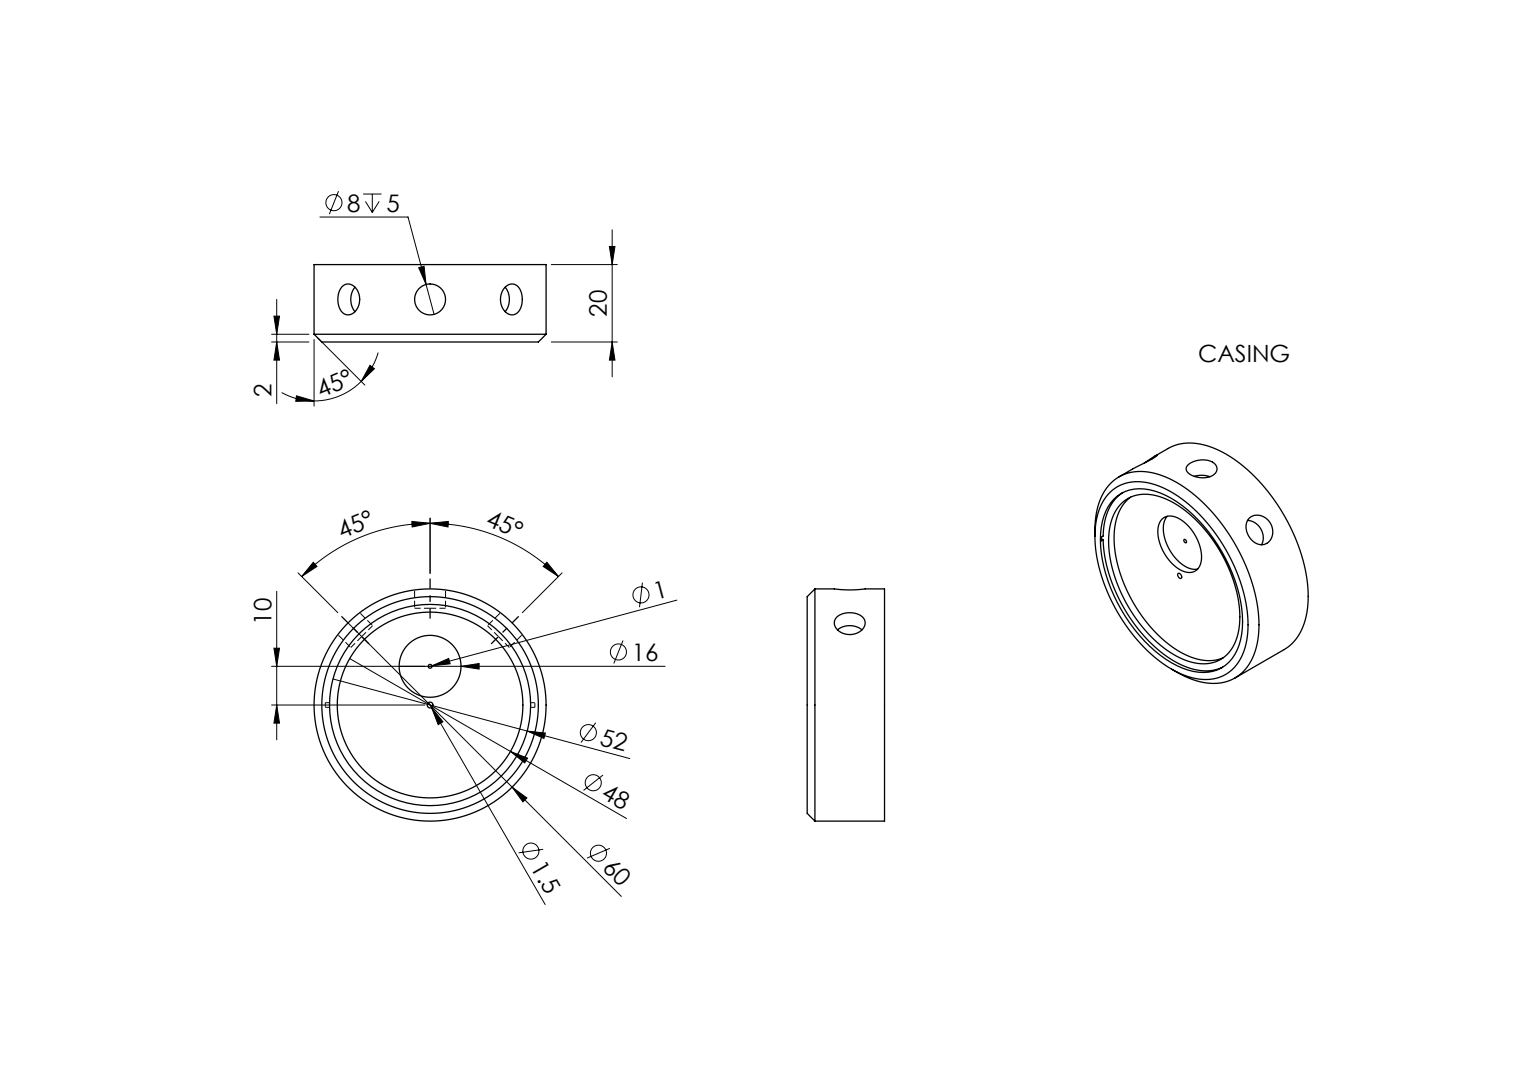
ISO-10303-21;
HEADER;
FILE_DESCRIPTION (('STEP AP214'),
    '1' );
FILE_NAME ('casing.step',
    '2026-10-26T11:20:31',
    ( '' ),
    ( '' ),
    'SwSTEP 2.0',
    'SolidWorks 2026',
    '' );
FILE_SCHEMA (( 'AUTOMOTIVE_DESIGN' ));
ENDSEC;

DATA;
#4=DIRECTION ( 'NONE',  ( 1.000000000000000000, 0.000000000000000000, 0.000000000000000000 ) ) ;
#15=CIRCLE ( 'NONE', #3506, 24.00000000000000355 ) ;
#17=CARTESIAN_POINT ( 'NONE',  ( 23.85222316637485562, 18.19536891688241198, 8.735393166554770161 ) ) ;
#23=EDGE_CURVE ( 'NONE', #3682, #3477, #99, .T. ) ;
#24=EDGE_CURVE ( 'NONE', #786, #1876, #1622, .T. ) ;
#31=CARTESIAN_POINT ( 'NONE',  ( -23.83674813237297130, 18.21571070649537916, 9.520895848189303123 ) ) ;
#33=CARTESIAN_POINT ( 'NONE',  ( -25.16843286583315376, -6.741346781237213648, 20.00001200000000168 ) ) ;
#38=CARTESIAN_POINT ( 'NONE',  ( 0.000000000000000000, 10.00000000000000000, 13.00000000000000178 ) ) ;
#40=CARTESIAN_POINT ( 'NONE',  ( 18.61772044889877264, 23.52449179749628883, 6.992605352578564748 ) ) ;
#41=CARTESIAN_POINT ( 'NONE',  ( -3.013274039476890653, 29.84885987243285399, 6.356496494711869616 ) ) ;
#43=MECHANICAL_DESIGN_GEOMETRIC_PRESENTATION_REPRESENTATION('',(#878),#2695);
#44=ORIENTED_EDGE ( 'NONE', *, *, #3267, .F. ) ;
#45=EDGE_CURVE ( 'NONE', #4134, #2111, #508, .T. ) ;
#57=LINE ( 'NONE', #2588, #2669 ) ;
#59=DIRECTION ( 'NONE',  ( 1.000000000000000000, 0.000000000000000000, 0.000000000000000000 ) ) ;
#64=CARTESIAN_POINT ( 'NONE',  ( 21.58020450303990145, 20.84134157445924274, 5.025533726064748130 ) ) ;
#69=ORIENTED_EDGE ( 'NONE', *, *, #4531, .T. ) ;
#72=AXIS2_PLACEMENT_3D ( 'NONE', #1710, #1001, #219 ) ;
#81=CARTESIAN_POINT ( 'NONE',  ( -18.19536891688249014, 23.85222316637480233, 9.264542937126581279 ) ) ;
#92=CARTESIAN_POINT ( 'NONE',  ( 23.23634976112698780, 18.97646788767667303, 6.355262957884884933 ) ) ;
#96=ORIENTED_EDGE ( 'NONE', *, *, #3914, .F. ) ;
#99=CIRCLE ( 'NONE', #4660, 24.00000000000000355 ) ;
#101=CYLINDRICAL_SURFACE ( 'NONE', #1304, 4.000000000000000000 ) ;
#105=EDGE_LOOP ( 'NONE', ( #1327, #855, #1076, #4619 ) ) ;
#107=CARTESIAN_POINT ( 'NONE',  ( -23.85222316637485207, 18.19536891688241553, 9.261144538644668245 ) ) ;
#108=CARTESIAN_POINT ( 'NONE',  ( 27.09999999999999787, -0.5999999999999998668, 19.59999999999999787 ) ) ;
#110=CARTESIAN_POINT ( 'NONE',  ( 27.09999999999999787, -0.5999999999999998668, 19.00000000000000000 ) ) ;
#111=CARTESIAN_POINT ( 'NONE',  ( 26.00000000000000355, 3.184081677783117796E-15, 19.59999999999999787 ) ) ;
#112=ADVANCED_FACE ( 'NONE', ( #3592 ), #4601, .T. ) ;
#115=CYLINDRICAL_SURFACE ( 'NONE', #1174, 24.00000000000000355 ) ;
#117=ORIENTED_EDGE ( 'NONE', *, *, #24, .F. ) ;
#122=AXIS2_PLACEMENT_3D ( 'NONE', #3838, #2369, #3476 ) ;
#125=ORIENTED_EDGE ( 'NONE', *, *, #1308, .T. ) ;
#126=EDGE_LOOP ( 'NONE', ( #4196, #3326, #979, #96 ) ) ;
#127=VERTEX_POINT ( 'NONE', #2121 ) ;
#131=VECTOR ( 'NONE', #4325, 1000.000000000000000 ) ;
#138=DIRECTION ( 'NONE',  ( 0.000000000000000000, -0.000000000000000000, -1.000000000000000000 ) ) ;
#143=DIRECTION ( 'NONE',  ( 1.000000000000000000, 0.000000000000000000, 0.000000000000000000 ) ) ;
#151=ORIENTED_EDGE ( 'NONE', *, *, #3914, .T. ) ;
#152=CARTESIAN_POINT ( 'NONE',  ( -25.99307600111999150, -0.5999999999999996447, 19.00000000000000000 ) ) ;
#157=CARTESIAN_POINT ( 'NONE',  ( -27.10000000000000497, -0.5999999999999998668, 19.00000000000000000 ) ) ;
#161=VECTOR ( 'NONE', #2341, 1000.000000000000000 ) ;
#162=CARTESIAN_POINT ( 'NONE',  ( -3.974466138550253103, 29.73560671006806899, 8.477544402765669673 ) ) ;
#164=PLANE ( 'NONE',  #630 ) ;
#169=EDGE_LOOP ( 'NONE', ( #4072, #812, #3404, #1028 ) ) ;
#171=EDGE_CURVE ( 'NONE', #2679, #1375, #2788, .T. ) ;
#174=PLANE ( 'NONE',  #3718 ) ;
#176=CIRCLE ( 'NONE', #3436, 4.000000000000000000 ) ;
#179=CARTESIAN_POINT ( 'NONE',  ( 0.000000000000000000, 10.00000000000000000, 15.00000000000000178 ) ) ;
#180=CARTESIAN_POINT ( 'NONE',  ( 8.000000000000000000, 10.00000000000000000, 15.00000000000000178 ) ) ;
#181=VERTEX_POINT ( 'NONE', #3190 ) ;
#185=CARTESIAN_POINT ( 'NONE',  ( -18.51903806033412891, 23.60202272616344743, 7.225073904196622543 ) ) ;
#187=CARTESIAN_POINT ( 'NONE',  ( -24.67207871933484498, 8.377607117416790317, 20.00001200000000523 ) ) ;
#189=EDGE_CURVE ( 'NONE', #2680, #3477, #311, .T. ) ;
#193=ADVANCED_FACE ( 'NONE', ( #334 ), #4702, .T. ) ;
#194=ORIENTED_EDGE ( 'NONE', *, *, #171, .F. ) ;
#195=CARTESIAN_POINT ( 'NONE',  ( 0.000000000000000000, 0.000000000000000000, 17.00000000000000000 ) ) ;
#204=EDGE_LOOP ( 'NONE', ( #2319, #1799, #3397, #669 ) ) ;
#208=CARTESIAN_POINT ( 'NONE',  ( 19.74742367678139132, 22.58509718322848769, 12.47015313278852844 ) ) ;
#212=CARTESIAN_POINT ( 'NONE',  ( -13.02991752792604707, 22.56362157461192908, 20.00001199999999812 ) ) ;
#217=ORIENTED_EDGE ( 'NONE', *, *, #23, .F. ) ;
#219=DIRECTION ( 'NONE',  ( 1.000000000000000000, 0.000000000000000000, 0.000000000000000000 ) ) ;
#220=DIRECTION ( 'NONE',  ( 0.000000000000000000, 0.000000000000000000, -1.000000000000000000 ) ) ;
#221=DIRECTION ( 'NONE',  ( 0.000000000000000000, 0.000000000000000000, 1.000000000000000000 ) ) ;
#224=CARTESIAN_POINT ( 'NONE',  ( 0.000000000000000000, 10.00000000000000000, 13.00000000000000178 ) ) ;
#226=FACE_OUTER_BOUND ( 'NONE', #2584, .T. ) ;
#227=EDGE_CURVE ( 'NONE', #883, #4468, #2767, .T. ) ;
#230=EDGE_CURVE ( 'NONE', #2552, #3925, #639, .T. ) ;
#236=DIRECTION ( 'NONE',  ( 0.000000000000000000, 0.000000000000000000, 1.000000000000000000 ) ) ;
#238=ORIENTED_EDGE ( 'NONE', *, *, #407, .F. ) ;
#239=EDGE_LOOP ( 'NONE', ( #2558, #2162, #259, #4443, #4049, #3898, #2909, #3068 ) ) ;
#240=FACE_OUTER_BOUND ( 'NONE', #4032, .T. ) ;
#241=DIRECTION ( 'NONE',  ( 0.000000000000000000, 0.000000000000000000, 1.000000000000000000 ) ) ;
#242=CARTESIAN_POINT ( 'NONE',  ( -3.403349963601461248, 25.83240171513484285, 20.00001200000000168 ) ) ;
#245=LINE ( 'NONE', #1716, #3549 ) ;
#247=VECTOR ( 'NONE', #3763, 1000.000000000000000 ) ;
#251=CARTESIAN_POINT ( 'NONE',  ( 18.51766120599535981, 23.60309964903844104, 10.77116693461329078 ) ) ;
#254=ADVANCED_FACE ( 'NONE', ( #2730 ), #1312, .F. ) ;
#259=ORIENTED_EDGE ( 'NONE', *, *, #1804, .T. ) ;
#262=FACE_OUTER_BOUND ( 'NONE', #1955, .T. ) ;
#265=SURFACE_SIDE_STYLE ('',( #3589 ) ) ;
#266=CARTESIAN_POINT ( 'NONE',  ( 27.09999999999999787, -0.5999999999999998668, 19.59999999999999787 ) ) ;
#268=AXIS2_PLACEMENT_3D ( 'NONE', #458, #2589, #3308 ) ;
#271=CARTESIAN_POINT ( 'NONE',  ( 0.2611446086310952874, 29.99999999999999645, 12.99999999999999112 ) ) ;
#272=ORIENTED_EDGE ( 'NONE', *, *, #761, .F. ) ;
#275=DIRECTION ( 'NONE',  ( 0.000000000000000000, 0.000000000000000000, 1.000000000000000000 ) ) ;
#276=CARTESIAN_POINT ( 'NONE',  ( 0.7500000000000001110, 0.000000000000000000, 17.00000000000000000 ) ) ;
#278=CARTESIAN_POINT ( 'NONE',  ( 17.67766952966372429, 17.67766952966365679, 8.999999999999992895 ) ) ;
#280=FACE_OUTER_BOUND ( 'NONE', #719, .T. ) ;
#283=EDGE_CURVE ( 'NONE', #741, #1146, #1292, .T. ) ;
#284=ORIENTED_EDGE ( 'NONE', *, *, #1600, .T. ) ;
#287=SHAPE_REPRESENTATION_RELATIONSHIP ( 'NONE' , 'NONE' ,  #1408, #2500 ) ;
#289=VERTEX_POINT ( 'NONE', #3854 ) ;
#290=DIRECTION ( 'NONE',  ( -1.000000000000000000, 0.000000000000000000, 0.000000000000000000 ) ) ;
#295=CARTESIAN_POINT ( 'NONE',  ( 1.289767132401806071, 29.97323123820465440, 12.79530979536915858 ) ) ;
#299=CARTESIAN_POINT ( 'NONE',  ( 25.99307600111999150, -0.5999999999999996447, 19.00000000000000000 ) ) ;
#300=CARTESIAN_POINT ( 'NONE',  ( 25.83240171513484285, -3.403349963601437267, 20.00001200000000168 ) ) ;
#301=CARTESIAN_POINT ( 'NONE',  ( -22.58496929628987360, 19.74756467586668762, 5.529782636833617815 ) ) ;
#305=VERTEX_POINT ( 'NONE', #1266 ) ;
#309=EDGE_CURVE ( 'NONE', #2969, #127, #2118, .T. ) ;
#311=LINE ( 'NONE', #4676, #943 ) ;
#315=CARTESIAN_POINT ( 'NONE',  ( 1.037548646792561202, 29.98316644498967776, 12.87206112426449955 ) ) ;
#318=AXIS2_PLACEMENT_3D ( 'NONE', #3626, #2522, #799 ) ;
#321=CARTESIAN_POINT ( 'NONE',  ( -26.00000000000000355, -1.592040838891558504E-15, 20.00000599999999906 ) ) ;
#332=ADVANCED_FACE ( 'NONE', ( #1356 ), #2431, .F. ) ;
#334=FACE_OUTER_BOUND ( 'NONE', #3811, .T. ) ;
#336=DIRECTION ( 'NONE',  ( 0.7071067811865487940, -0.7071067811865463515, 0.000000000000000000 ) ) ;
#338=CARTESIAN_POINT ( 'NONE',  ( 0.000000000000000000, 0.000000000000000000, 17.00000000000000000 ) ) ;
#339=CARTESIAN_POINT ( 'NONE',  ( 2.445228802079471908, 29.90098466201939331, 5.823513562339502236 ) ) ;
#340=AXIS2_PLACEMENT_3D ( 'NONE', #4186, #2765, #968 ) ;
#343=CARTESIAN_POINT ( 'NONE',  ( 22.99946665860936079, 19.26288713789788076, 12.01444203287436174 ) ) ;
#350=ORIENTED_EDGE ( 'NONE', *, *, #987, .F. ) ;
#351=EDGE_LOOP ( 'NONE', ( #3080, #1048, #1376, #4284 ) ) ;
#353=DIRECTION ( 'NONE',  ( 0.000000000000000000, 0.000000000000000000, 1.000000000000000000 ) ) ;
#354=ORIENTED_EDGE ( 'NONE', *, *, #189, .T. ) ;
#360=VECTOR ( 'NONE', #3662, 1000.000000000000000 ) ;
#363=EDGE_CURVE ( 'NONE', #3116, #786, #4257, .T. ) ;
#365=CIRCLE ( 'NONE', #72, 0.5000000000000001110 ) ;
#368=AXIS2_PLACEMENT_3D ( 'NONE', #485, #3386, #138 ) ;
#373=DIRECTION ( 'NONE',  ( 0.000000000000000000, 0.000000000000000000, 1.000000000000000000 ) ) ;
#383=EDGE_LOOP ( 'NONE', ( #2433, #2317, #125, #4259 ) ) ;
#388=CARTESIAN_POINT ( 'NONE',  ( 23.60202272616350783, 18.51903806033405075, 7.225073904196623431 ) ) ;
#390=EDGE_CURVE ( 'NONE', #3925, #1876, #667, .T. ) ;
#392=ADVANCED_FACE ( 'NONE', ( #280 ), #3556, .F. ) ;
#394=ORIENTED_EDGE ( 'NONE', *, *, #1600, .F. ) ;
#401=ORIENTED_EDGE ( 'NONE', *, *, #3956, .F. ) ;
#405=FACE_OUTER_BOUND ( 'NONE', #3345, .T. ) ;
#406=DIRECTION ( 'NONE',  ( -0.000000000000000000, -0.000000000000000000, 1.000000000000000000 ) ) ;
#407=EDGE_CURVE ( 'NONE', #4099, #956, #3629, .T. ) ;
#409=AXIS2_PLACEMENT_3D ( 'NONE', #952, #3826, #4194 ) ;
#414=CARTESIAN_POINT ( 'NONE',  ( 22.43029000766442493, 19.92335677698576291, 5.404794703904384434 ) ) ;
#417=EDGE_LOOP ( 'NONE', ( #3095, #2362, #3318, #3383, #3652 ) ) ;
#421=AXIS2_PLACEMENT_3D ( 'NONE', #2479, #3250, #1065 ) ;
#431=CARTESIAN_POINT ( 'NONE',  ( -23.77376218378628181, 18.29783893517727478, 10.03754308049874311 ) ) ;
#433=CARTESIAN_POINT ( 'NONE',  ( 26.00000000000000355, 1.592040838891558898E-15, 20.00000599999999906 ) ) ;
#436=CYLINDRICAL_SURFACE ( 'NONE', #571, 3.999999999999998224 ) ;
#452=ORIENTED_EDGE ( 'NONE', *, *, #2236, .F. ) ;
#458=CARTESIAN_POINT ( 'NONE',  ( 0.000000000000000000, 10.00000000000000000, 15.00000000000000178 ) ) ;
#462=CARTESIAN_POINT ( 'NONE',  ( -27.10000000000000497, -0.5999999999999998668, 19.59999999999999787 ) ) ;
#465=CARTESIAN_POINT ( 'NONE',  ( 0.000000000000000000, 0.000000000000000000, 17.99999999999998579 ) ) ;
#470=CARTESIAN_POINT ( 'NONE',  ( -17.67766952966371719, 17.67766952966366389, 8.999999999999992895 ) ) ;
#471=CARTESIAN_POINT ( 'NONE',  ( -27.10000000000000497, -0.5999999999999998668, 19.00000000000000000 ) ) ;
#476=ORIENTED_EDGE ( 'NONE', *, *, #1700, .F. ) ;
#480=CARTESIAN_POINT ( 'NONE',  ( -18.61790092284054410, 23.52435923723752609, 11.00811882721853152 ) ) ;
#485=CARTESIAN_POINT ( 'NONE',  ( -27.10000000000000497, 0.6000000000000000888, 19.59999999999999787 ) ) ;
#490=CARTESIAN_POINT ( 'NONE',  ( -1.774938052278379752, 29.94842879300231075, 5.405792698933810314 ) ) ;
#500=ORIENTED_EDGE ( 'NONE', *, *, #1073, .F. ) ;
#501=ORIENTED_EDGE ( 'NONE', *, *, #866, .F. ) ;
#506=CARTESIAN_POINT ( 'NONE',  ( 0.000000000000000000, 0.000000000000000000, 17.00000000000000000 ) ) ;
#508=LINE ( 'NONE', #3408, #1317 ) ;
#513=ORIENTED_EDGE ( 'NONE', *, *, #1744, .T. ) ;
#519=CARTESIAN_POINT ( 'NONE',  ( -18.29773070266338664, 23.77384460521234288, 7.963596978677149885 ) ) ;
#533=ORIENTED_EDGE ( 'NONE', *, *, #4639, .F. ) ;
#534=DIRECTION ( 'NONE',  ( 0.000000000000000000, 1.000000000000000000, 0.000000000000000000 ) ) ;
#535=PLANE ( 'NONE',  #4253 ) ;
#536=FACE_BOUND ( 'NONE', #2532, .T. ) ;
#537=ORIENTED_EDGE ( 'NONE', *, *, #1804, .F. ) ;
#539=VECTOR ( 'NONE', #2025, 1000.000000000000000 ) ;
#540=CARTESIAN_POINT ( 'NONE',  ( 18.19536891688249369, 23.85222316637479523, 8.999999999999992895 ) ) ;
#547=DIRECTION ( 'NONE',  ( 1.000000000000000000, 0.000000000000000000, 0.000000000000000000 ) ) ;
#549=EDGE_LOOP ( 'NONE', ( #476, #1269 ) ) ;
#550=ORIENTED_EDGE ( 'NONE', *, *, #3857, .F. ) ;
#561=ORIENTED_EDGE ( 'NONE', *, *, #1435, .T. ) ;
#567=CARTESIAN_POINT ( 'NONE',  ( -18.61638332444503519, 23.52555220673917447, 6.995423750305947763 ) ) ;
#569=CARTESIAN_POINT ( 'NONE',  ( -26.00000000000000355, -1.592040838891558504E-15, 20.00000599999999906 ) ) ;
#571=AXIS2_PLACEMENT_3D ( 'NONE', #3387, #3314, #1154 ) ;
#585=DIRECTION ( 'NONE',  ( 0.000000000000000000, 0.000000000000000000, 1.000000000000000000 ) ) ;
#586=CARTESIAN_POINT ( 'NONE',  ( 3.469446951953614189E-15, 30.00000000000000355, 8.999999999999992895 ) ) ;
#591=CARTESIAN_POINT ( 'NONE',  ( -14.84924240491753089, 20.50609665440985552, 8.999999999999992895 ) ) ;
#593=CARTESIAN_POINT ( 'NONE',  ( 19.25985638980603554, 23.00200370561274354, 12.01100206247544300 ) ) ;
#594=DIRECTION ( 'NONE',  ( -1.000000000000000000, -0.000000000000000000, -0.000000000000000000 ) ) ;
#595=CARTESIAN_POINT ( 'NONE',  ( -21.58204166899923138, 20.83941891177991224, 5.025993266704736229 ) ) ;
#602=CARTESIAN_POINT ( 'NONE',  ( -27.10000000000000497, 0.6000000000000000888, 19.59999999999999787 ) ) ;
#606=STYLED_ITEM('',(#4736),#2883);
#611=EDGE_CURVE ( 'NONE', #4468, #4460, #1182, .T. ) ;
#616=CARTESIAN_POINT ( 'NONE',  ( -2.007411586324088226, 29.93355017142139118, 12.46960170373642640 ) ) ;
#618=CARTESIAN_POINT ( 'NONE',  ( -23.85222316637485562, 18.19536891688241198, 8.999999999999992895 ) ) ;
#623=ORIENTED_EDGE ( 'NONE', *, *, #3700, .F. ) ;
#624=ADVANCED_FACE ( 'NONE', ( #2648 ), #2287, .T. ) ;
#629=CARTESIAN_POINT ( 'NONE',  ( 8.377607117416813409, 24.67207871933482366, 20.00001200000000523 ) ) ;
#630=AXIS2_PLACEMENT_3D ( 'NONE', #850, #2727, #2290 ) ;
#634=CARTESIAN_POINT ( 'NONE',  ( 3.796098697355190676, 29.75902942016942987, 7.712254142552557923 ) ) ;
#639=CIRCLE ( 'NONE', #3339, 26.00000000000000355 ) ;
#640=DIRECTION ( 'NONE',  ( 0.000000000000000000, 0.000000000000000000, -1.000000000000000000 ) ) ;
#644=DIRECTION ( 'NONE',  ( 1.000000000000000000, 0.000000000000000000, 0.000000000000000000 ) ) ;
#647=CIRCLE ( 'NONE', #3292, 26.00000000000000355 ) ;
#648=CARTESIAN_POINT ( 'NONE',  ( 27.09999999999999787, 0.6000000000000000888, 19.59999999999999787 ) ) ;
#649=DIRECTION ( 'NONE',  ( 0.000000000000000000, 0.000000000000000000, -1.000000000000000000 ) ) ;
#650=CIRCLE ( 'NONE', #4445, 26.00000000000000355 ) ;
#651=( LENGTH_UNIT ( ) NAMED_UNIT ( * ) SI_UNIT ( .MILLI., .METRE. ) );
#656=( GEOMETRIC_REPRESENTATION_CONTEXT ( 3 ) GLOBAL_UNCERTAINTY_ASSIGNED_CONTEXT ( ( #1169 ) ) GLOBAL_UNIT_ASSIGNED_CONTEXT ( ( #3518, #1074, #4331 ) ) REPRESENTATION_CONTEXT ( 'NONE', 'WORKASPACE' ) );
#657=( NAMED_UNIT ( * ) SI_UNIT ( $, .STERADIAN. ) SOLID_ANGLE_UNIT ( ) );
#665=CARTESIAN_POINT ( 'NONE',  ( -23.52449179749635277, 18.61772044889870159, 6.992605352578565636 ) ) ;
#667=LINE ( 'NONE', #1046, #131 ) ;
#669=ORIENTED_EDGE ( 'NONE', *, *, #1744, .F. ) ;
#674=CARTESIAN_POINT ( 'NONE',  ( 24.00000000000000355, 0.000000000000000000, 17.00000000000000000 ) ) ;
#679=DIRECTION ( 'NONE',  ( 1.000000000000000000, 0.000000000000000000, 0.000000000000000000 ) ) ;
#681=CYLINDRICAL_SURFACE ( 'NONE', #1102, 0.7500000000000001110 ) ;
#694=ORIENTED_EDGE ( 'NONE', *, *, #4339, .F. ) ;
#698=VECTOR ( 'NONE', #1121, 1000.000000000000000 ) ;
#703=LINE ( 'NONE', #1079, #900 ) ;
#704=CARTESIAN_POINT ( 'NONE',  ( 3.872997316437435167, 29.74899170013632954, 7.966596725458382267 ) ) ;
#705=CIRCLE ( 'NONE', #1311, 0.7500000000000001110 ) ;
#707=VECTOR ( 'NONE', #1175, 1000.000000000000000 ) ;
#708=B_SPLINE_CURVE_WITH_KNOTS ( 'NONE', 3,
 ( #3293, #846, #2286, #1159, #3745, #490, #823, #2264, #4490, #41, #2216, #1864, #3670, #1604, #4165, #162, #3129, #3463, #2745, #2796, #4252, #2351, #4610, #898, #2425, #2037, #3823, #616, #2328, #1989, #993, #948, #2770, #3438 ),
 .UNSPECIFIED., .F., .F.,
 ( 4, 2, 2, 2, 2, 2, 2, 2, 2, 2, 2, 2, 2, 2, 2, 2, 4 ),
 ( 0.000000000000000000, 0.0007824850735655043557, 0.001564970147131008711, 0.002347455220696513176, 0.003129940294262017423, 0.003912425367827521670, 0.004694910441393026351, 0.005477395514958530165, 0.006259880588524034846, 0.007042365662089539527, 0.007824850735655043341, 0.008607335809220547154, 0.009389820882786052703, 0.01017230595635155652, 0.01095479102991706033, 0.01173727610348256588, 0.01251976117704806969 ),
 .UNSPECIFIED. ) ;
#712=CARTESIAN_POINT ( 'NONE',  ( -27.10000000000000497, -0.5999999999999998668, 19.00000000000000000 ) ) ;
#719=EDGE_LOOP ( 'NONE', ( #3325, #1461, #3259, #694 ) ) ;
#721=CARTESIAN_POINT ( 'NONE',  ( 3.403349963601422168, 25.83240171513484285, 20.00001200000000523 ) ) ;
#722=EDGE_CURVE ( 'NONE', #4523, #3514, #2026, .T. ) ;
#724=EDGE_CURVE ( 'NONE', #2854, #2731, #4586, .T. ) ;
#729=AXIS2_PLACEMENT_3D ( 'NONE', #506, #221, #3815 ) ;
#730=DIRECTION ( 'NONE',  ( 1.000000000000000000, 0.000000000000000000, -0.000000000000000000 ) ) ;
#731=CIRCLE ( 'NONE', #3389, 8.000000000000000000 ) ;
#732=CYLINDRICAL_SURFACE ( 'NONE', #3891, 0.7500000000000001110 ) ;
#735=VECTOR ( 'NONE', #2831, 1000.000000000000000 ) ;
#740=DIRECTION ( 'NONE',  ( 1.000000000000000000, 0.000000000000000000, 0.000000000000000000 ) ) ;
#741=VERTEX_POINT ( 'NONE', #2403 ) ;
#747=EDGE_LOOP ( 'NONE', ( #2220, #2706, #1118, #1381 ) ) ;
#749=EDGE_CURVE ( 'NONE', #1146, #1098, #2012, .T. ) ;
#750=VECTOR ( 'NONE', #3405, 1000.000000000000000 ) ;
#761=EDGE_CURVE ( 'NONE', #4484, #1375, #3922, .T. ) ;
#769=CARTESIAN_POINT ( 'NONE',  ( -18.84808613845423508, 23.34033764136069422, 11.44520879210846687 ) ) ;
#770=DIRECTION ( 'NONE',  ( -0.000000000000000000, -0.000000000000000000, -1.000000000000000000 ) ) ;
#771=CARTESIAN_POINT ( 'NONE',  ( 15.85973458909327505, -20.67279826512041296, 20.00001199999999457 ) ) ;
#772=ORIENTED_EDGE ( 'NONE', *, *, #1404, .T. ) ;
#775=CARTESIAN_POINT ( 'NONE',  ( -8.000000000000000000, 10.00000000000000178, 15.00000000000000178 ) ) ;
#778=EDGE_CURVE ( 'NONE', #956, #1513, #731, .T. ) ;
#779=DIRECTION ( 'NONE',  ( -0.000000000000000000, -0.000000000000000000, 1.000000000000000000 ) ) ;
#786=VERTEX_POINT ( 'NONE', #4232 ) ;
#789=DIRECTION ( 'NONE',  ( -0.000000000000000000, -0.000000000000000000, 1.000000000000000000 ) ) ;
#793=EDGE_LOOP ( 'NONE', ( #1095, #3584 ) ) ;
#794=AXIS2_PLACEMENT_3D ( 'NONE', #465, #2986, #2671 ) ;
#796=DIRECTION ( 'NONE',  ( 1.000000000000000000, 0.000000000000000000, 0.000000000000000000 ) ) ;
#797=AXIS2_PLACEMENT_3D ( 'NONE', #4318, #1787, #3597 ) ;
#799=DIRECTION ( 'NONE',  ( 1.000000000000000000, 0.000000000000000000, 0.000000000000000000 ) ) ;
#802=ORIENTED_EDGE ( 'NONE', *, *, #1661, .F. ) ;
#811=ORIENTED_EDGE ( 'NONE', *, *, #4287, .T. ) ;
#812=ORIENTED_EDGE ( 'NONE', *, *, #1517, .F. ) ;
#814=CARTESIAN_POINT ( 'NONE',  ( -21.40213195504977861, 21.02424009228906243, 12.99981531858142425 ) ) ;
#817=CARTESIAN_POINT ( 'NONE',  ( -25.99307600111999150, 0.5999999999999998668, 19.59999999999999787 ) ) ;
#822=CARTESIAN_POINT ( 'NONE',  ( 18.19536891688249369, 23.85222316637479523, 8.999999999999992895 ) ) ;
#823=CARTESIAN_POINT ( 'NONE',  ( -2.004590926901224535, 29.93374515888019971, 5.528701699505815803 ) ) ;
#830=DIRECTION ( 'NONE',  ( 1.000000000000000000, 0.000000000000000000, 0.000000000000000000 ) ) ;
#840=CARTESIAN_POINT ( 'NONE',  ( -23.00200370561280749, 19.25985638980596093, 12.01100206247544300 ) ) ;
#843=AXIS2_PLACEMENT_3D ( 'NONE', #2460, #2508, #3928 ) ;
#846=CARTESIAN_POINT ( 'NONE',  ( -0.2646063747045178660, 30.00000000000000000, 4.999999999999992895 ) ) ;
#850=CARTESIAN_POINT ( 'NONE',  ( -27.10000000000000497, -0.5999999999999998668, 19.59999999999999787 ) ) ;
#855=ORIENTED_EDGE ( 'NONE', *, *, #2538, .T. ) ;
#866=EDGE_CURVE ( 'NONE', #4468, #883, #1530, .T. ) ;
#867=DIRECTION ( 'NONE',  ( 0.000000000000000000, 0.000000000000000000, 1.000000000000000000 ) ) ;
#869=ORIENTED_EDGE ( 'NONE', *, *, #722, .T. ) ;
#871=B_SPLINE_CURVE_WITH_KNOTS ( 'NONE', 3,
 ( #540, #1305, #4536, #1281, #4211, #251, #1652, #1969, #1353, #593, #3416, #208, #2011, #2724, #3109, #2376, #3847, #1330, #4231, #3870, #1698, #1085, #4341, #3986, #343, #1745, #2911, #4635, #2104, #2520, #1722, #3624, #2497, #3529 ),
 .UNSPECIFIED., .F., .F.,
 ( 4, 2, 2, 2, 2, 2, 2, 2, 2, 2, 2, 2, 2, 2, 2, 2, 4 ),
 ( 0.01251975318912558477, 0.01330204881184919585, 0.01408434443457280694, 0.01486664005729641802, 0.01564893568002002910, 0.01643123130274364019, 0.01721352692546725127, 0.01799582254819086236, 0.01877811817091447344, 0.01956041379363808452, 0.02034270941636169561, 0.02112500503908530669, 0.02190730066180891430, 0.02268959628453252539, 0.02347189190725613647, 0.02425418752997974756, 0.02503648315270335864 ),
 .UNSPECIFIED. ) ;
#875=CARTESIAN_POINT ( 'NONE',  ( -20.46659425767094120, 21.93593546006592732, 5.128325996195414405 ) ) ;
#878=STYLED_ITEM ( 'NONE', ( #1424 ), #2500 ) ;
#879=DIRECTION ( 'NONE',  ( 0.000000000000000000, -1.000000000000000000, 0.000000000000000000 ) ) ;
#882=ORIENTED_EDGE ( 'NONE', *, *, #3578, .T. ) ;
#883=VERTEX_POINT ( 'NONE', #433 ) ;
#884=CARTESIAN_POINT ( 'NONE',  ( 0.000000000000000000, 0.000000000000000000, 20.00000000000000000 ) ) ;
#891=ADVANCED_FACE ( 'NONE', ( #1883 ), #3893, .F. ) ;
#893=FACE_BOUND ( 'NONE', #793, .T. ) ;
#897=EDGE_CURVE ( 'NONE', #1997, #4134, #2797, .T. ) ;
#898=CARTESIAN_POINT ( 'NONE',  ( -3.180741987853693331, 29.83126030492351788, 11.43940974718624837 ) ) ;
#900=VECTOR ( 'NONE', #4268, 1000.000000000000000 ) ;
#902=AXIS2_PLACEMENT_3D ( 'NONE', #2490, #3214, #3962 ) ;
#903=DIRECTION ( 'NONE',  ( -0.7071067811865487940, -0.7071067811865463515, 0.000000000000000000 ) ) ;
#906=VERTEX_POINT ( 'NONE', #3530 ) ;
#907=VERTEX_POINT ( 'NONE', #276 ) ;
#910=CARTESIAN_POINT ( 'NONE',  ( 3.959305739469038251E-15, 30.00000000000000355, 12.99999999999999289 ) ) ;
#913=DIRECTION ( 'NONE',  ( 0.000000000000000000, 0.000000000000000000, -1.000000000000000000 ) ) ;
#914=ADVANCED_FACE ( 'NONE', ( #4637 ), #2820, .F. ) ;
#930=CARTESIAN_POINT ( 'NONE',  ( -30.00000000000004974, 29.99999999999995737, 8.999999999999992895 ) ) ;
#943=VECTOR ( 'NONE', #1692, 1000.000000000000000 ) ;
#944=DIRECTION ( 'NONE',  ( 0.7071067811865487940, -0.7071067811865463515, 0.000000000000000000 ) ) ;
#948=CARTESIAN_POINT ( 'NONE',  ( -0.5265545572341292502, 29.99647701088549923, 12.97381592328244082 ) ) ;
#950=CIRCLE ( 'NONE', #3602, 8.000000000000000000 ) ;
#952=CARTESIAN_POINT ( 'NONE',  ( -17.67766952966371719, 17.67766952966366389, 8.999999999999992895 ) ) ;
#953=DIRECTION ( 'NONE',  ( 0.7071067811865462405, 0.7071067811865487940, 0.000000000000000000 ) ) ;
#956=VERTEX_POINT ( 'NONE', #1781 ) ;
#965=ORIENTED_EDGE ( 'NONE', *, *, #4384, .T. ) ;
#968=DIRECTION ( 'NONE',  ( 1.000000000000000000, 0.000000000000000000, -0.000000000000000000 ) ) ;
#974=EDGE_CURVE ( 'NONE', #127, #2969, #1720, .T. ) ;
#977=CARTESIAN_POINT ( 'NONE',  ( -27.99999999999999645, 0.000000000000000000, 20.00000000000000000 ) ) ;
#978=CARTESIAN_POINT ( 'NONE',  ( -26.00000000000000000, 1.701696020694461131, 20.00001199999999812 ) ) ;
#979=ORIENTED_EDGE ( 'NONE', *, *, #4589, .T. ) ;
#984=FILL_AREA_STYLE ('',( #1004 ) ) ;
#987=EDGE_CURVE ( 'NONE', #2090, #3682, #1802, .T. ) ;
#988=DIRECTION ( 'NONE',  ( 1.000000000000000000, 0.000000000000000000, 0.000000000000000000 ) ) ;
#991=CARTESIAN_POINT ( 'NONE',  ( 3.593167859435787204, 29.78421435497087444, 10.77704851721127177 ) ) ;
#993=CARTESIAN_POINT ( 'NONE',  ( -1.039771317798496408, 29.98307469845295969, 12.87134967428165666 ) ) ;
#994=CARTESIAN_POINT ( 'NONE',  ( -27.10000000000000497, -0.5999999999999998668, 19.59999999999999787 ) ) ;
#1001=DIRECTION ( 'NONE',  ( 0.000000000000000000, 0.000000000000000000, 1.000000000000000000 ) ) ;
#1004=FILL_AREA_STYLE_COLOUR ( '', #1477 ) ;
#1005=CARTESIAN_POINT ( 'NONE',  ( -6.741346781237239405, 25.16843286583313954, 20.00001200000000168 ) ) ;
#1009=CARTESIAN_POINT ( 'NONE',  ( 1.042990544031788813, 29.98297896446152322, 5.129385753419673399 ) ) ;
#1014=DIRECTION ( 'NONE',  ( -1.000000000000000000, 0.000000000000000000, 0.000000000000000000 ) ) ;
#1016=CARTESIAN_POINT ( 'NONE',  ( 13.02991752792604174, -22.56362157461193263, 20.00001200000000168 ) ) ;
#1017=CARTESIAN_POINT ( 'NONE',  ( -23.85222316637485562, 18.19536891688241909, 8.738792385868096702 ) ) ;
#1028=ORIENTED_EDGE ( 'NONE', *, *, #1435, .F. ) ;
#1031=CYLINDRICAL_SURFACE ( 'NONE', #3057, 0.5000000000000001110 ) ;
#1033=CARTESIAN_POINT ( 'NONE',  ( 3.472993751331377332, 29.79865100271689471, 6.998343904161816731 ) ) ;
#1034=EDGE_CURVE ( 'NONE', #181, #289, #4312, .T. ) ;
#1035=EDGE_CURVE ( 'NONE', #2995, #4460, #2546, .T. ) ;
#1042=CARTESIAN_POINT ( 'NONE',  ( 19.58805710660147170, -17.18149551509900519, 20.00001200000000523 ) ) ;
#1046=CARTESIAN_POINT ( 'NONE',  ( -27.10000000000000497, -0.5999999999999998668, 19.00000000000000000 ) ) ;
#1048=ORIENTED_EDGE ( 'NONE', *, *, #4587, .T. ) ;
#1049=CARTESIAN_POINT ( 'NONE',  ( -27.10000000000000497, 0.6000000000000000888, 19.59999999999999787 ) ) ;
#1052=ORIENTED_EDGE ( 'NONE', *, *, #749, .F. ) ;
#1055=FACE_OUTER_BOUND ( 'NONE', #1448, .T. ) ;
#1064=LINE ( 'NONE', #2194, #2300 ) ;
#1065=DIRECTION ( 'NONE',  ( 1.000000000000000000, 0.000000000000000000, 0.000000000000000000 ) ) ;
#1069=AXIS2_PLACEMENT_3D ( 'NONE', #4115, #2357, #1284 ) ;
#1073=EDGE_CURVE ( 'NONE', #3706, #3924, #2200, .T. ) ;
#1074=( NAMED_UNIT ( * ) PLANE_ANGLE_UNIT ( ) SI_UNIT ( $, .RADIAN. ) );
#1076=ORIENTED_EDGE ( 'NONE', *, *, #2773, .F. ) ;
#1077=CARTESIAN_POINT ( 'NONE',  ( 15.85973458909325728, 20.67279826512042362, 20.00001200000000168 ) ) ;
#1079=CARTESIAN_POINT ( 'NONE',  ( -27.10000000000000497, 0.6000000000000000888, 19.00000000000000000 ) ) ;
#1085=CARTESIAN_POINT ( 'NONE',  ( 22.42982507849026064, 19.92389804225921068, 12.59566700906149173 ) ) ;
#1088=DIRECTION ( 'NONE',  ( -0.000000000000000000, -0.000000000000000000, 1.000000000000000000 ) ) ;
#1093=PLANE ( 'NONE',  #3890 ) ;
#1095=ORIENTED_EDGE ( 'NONE', *, *, #3106, .F. ) ;
#1098=VERTEX_POINT ( 'NONE', #1901 ) ;
#1102=AXIS2_PLACEMENT_3D ( 'NONE', #3571, #2494, #4338 ) ;
#1104=DIRECTION ( 'NONE',  ( -0.000000000000000000, -0.000000000000000000, -1.000000000000000000 ) ) ;
#1107=AXIS2_PLACEMENT_3D ( 'NONE', #4548, #3049, #2713 ) ;
#1109=SHAPE_DEFINITION_REPRESENTATION ( #3051, #1408 ) ;
#1118=ORIENTED_EDGE ( 'NONE', *, *, #2395, .T. ) ;
#1121=DIRECTION ( 'NONE',  ( 0.7071067811865456854, 8.659560562354910671E-17, -0.7071067811865493491 ) ) ;
#1125=CARTESIAN_POINT ( 'NONE',  ( 25.99307600111999150, 0.6000000000000000888, 20.00001200000000168 ) ) ;
#1128=CARTESIAN_POINT ( 'NONE',  ( -22.56362157461193618, -13.02991752792603641, 20.00001200000000168 ) ) ;
#1135=AXIS2_PLACEMENT_3D ( 'NONE', #3491, #236, #3136 ) ;
#1137=CARTESIAN_POINT ( 'NONE',  ( 18.84534098761077914, 23.34254382248196791, 6.559627254860783019 ) ) ;
#1143=CARTESIAN_POINT ( 'NONE',  ( 0.000000000000000000, 0.000000000000000000, 17.00000000000000000 ) ) ;
#1146=VERTEX_POINT ( 'NONE', #3349 ) ;
#1147=ORIENTED_EDGE ( 'NONE', *, *, #45, .T. ) ;
#1149=LINE ( 'NONE', #1125, #4279 ) ;
#1151=CARTESIAN_POINT ( 'NONE',  ( -19.75109744359749797, 22.58188871325890901, 12.47298490618377897 ) ) ;
#1152=CARTESIAN_POINT ( 'NONE',  ( -17.18149551509900519, -19.58805710660146104, 20.00001200000000523 ) ) ;
#1154=DIRECTION ( 'NONE',  ( 0.7071067811865462405, 0.7071067811865487940, 0.000000000000000000 ) ) ;
#1155=ADVANCED_FACE ( 'NONE', ( #1512 ), #3400, .T. ) ;
#1158=CARTESIAN_POINT ( 'NONE',  ( 18.97448886297823378, 23.23798364781081816, 6.357861838490106443 ) ) ;
#1159=CARTESIAN_POINT ( 'NONE',  ( -1.036406108997123487, 29.98318460927812268, 5.127803451112008304 ) ) ;
#1162=ORIENTED_EDGE ( 'NONE', *, *, #4064, .T. ) ;
#1169=UNCERTAINTY_MEASURE_WITH_UNIT (LENGTH_MEASURE( 1.000000000000000082E-05 ), #3518, 'distance_accuracy_value', 'NONE');
#1170=LINE ( 'NONE', #4456, #750 ) ;
#1174=AXIS2_PLACEMENT_3D ( 'NONE', #4112, #1891, #2647 ) ;
#1175=DIRECTION ( 'NONE',  ( -0.000000000000000000, -0.000000000000000000, -1.000000000000000000 ) ) ;
#1179=FACE_OUTER_BOUND ( 'NONE', #126, .T. ) ;
#1182=LINE ( 'NONE', #1921, #2934 ) ;
#1183=ORIENTED_EDGE ( 'NONE', *, *, #3553, .T. ) ;
#1189=CARTESIAN_POINT ( 'NONE',  ( 23.83633674995677509, 18.21624787168408588, 8.475268202211099222 ) ) ;
#1193=ORIENTED_EDGE ( 'NONE', *, *, #283, .F. ) ;
#1197=CARTESIAN_POINT ( 'NONE',  ( -30.00000000000000355, 0.000000000000000000, 17.99999999999998579 ) ) ;
#1209=DIRECTION ( 'NONE',  ( 1.000000000000000000, 0.000000000000000000, 0.000000000000000000 ) ) ;
#1210=CARTESIAN_POINT ( 'NONE',  ( 18.19536891688249369, 23.85222316637479523, 8.999999999999992895 ) ) ;
#1214=ORIENTED_EDGE ( 'NONE', *, *, #866, .T. ) ;
#1215=ADVANCED_FACE ( 'NONE', ( #4071 ), #101, .F. ) ;
#1219=EDGE_LOOP ( 'NONE', ( #537, #3228, #4593, #1147 ) ) ;
#1224=CARTESIAN_POINT ( 'NONE',  ( 3.469446951953614189E-15, 30.00000000000000355, 4.999999999999992006 ) ) ;
#1228=B_SPLINE_CURVE_WITH_KNOTS ( 'NONE', 3,
 ( #3649, #17, #1189, #2549, #4014, #388, #2215, #3668, #92, #2940, #4061, #1890, #414, #3269, #2985, #64, #2962, #4390, #1458, #3291, #4416, #2623, #3340, #2913, #1795, #1158, #1137, #40, #1482, #4438, #1436, #2890, #4087, #822 ),
 .UNSPECIFIED., .F., .F.,
 ( 4, 2, 2, 2, 2, 2, 2, 2, 2, 2, 2, 2, 2, 2, 2, 2, 4 ),
 ( 0.000000000000000000, 0.0007824845743203473133, 0.001564969148640694627, 0.002347453722961044108, 0.003129938297281393590, 0.003912422871601742638, 0.004694907445922092554, 0.005477392020242441602, 0.006259876594562790650, 0.007042361168883141433, 0.007824845743203490481, 0.008607330317523840396, 0.009389814891844192046, 0.01017229946616454196, 0.01095478404048489014, 0.01173726861480523832, 0.01251975318912558477 ),
 .UNSPECIFIED. ) ;
#1234=DIRECTION ( 'NONE',  ( 0.000000000000000000, 0.000000000000000000, 1.000000000000000000 ) ) ;
#1253=PLANE ( 'NONE',  #1884 ) ;
#1255=ORIENTED_EDGE ( 'NONE', *, *, #4587, .F. ) ;
#1257=AXIS2_PLACEMENT_3D ( 'NONE', #586, #2305, #3768 ) ;
#1258=LINE ( 'NONE', #2696, #2081 ) ;
#1259=DIRECTION ( 'NONE',  ( 0.000000000000000000, 0.000000000000000000, 1.000000000000000000 ) ) ;
#1260=EDGE_CURVE ( 'NONE', #883, #4187, #1640, .T. ) ;
#1262=CARTESIAN_POINT ( 'NONE',  ( -19.26183863435818822, 23.00034469605611775, 5.986743120287543185 ) ) ;
#1266=CARTESIAN_POINT ( 'NONE',  ( 25.99307600111999150, 0.5999999999999998668, 19.59999999999999787 ) ) ;
#1269=ORIENTED_EDGE ( 'NONE', *, *, #2002, .F. ) ;
#1271=CARTESIAN_POINT ( 'NONE',  ( 20.50609665440990526, 14.84924240491746517, 8.999999999999992895 ) ) ;
#1274=ORIENTED_EDGE ( 'NONE', *, *, #2139, .F. ) ;
#1280=ADVANCED_FACE ( 'NONE', ( #3860 ), #4649, .T. ) ;
#1281=CARTESIAN_POINT ( 'NONE',  ( 18.29783893517735294, 23.77376218378621431, 10.03754308049874133 ) ) ;
#1282=DIRECTION ( 'NONE',  ( 0.000000000000000000, 1.000000000000000000, 0.000000000000000000 ) ) ;
#1283=VECTOR ( 'NONE', #1924, 1000.000000000000000 ) ;
#1284=DIRECTION ( 'NONE',  ( -1.000000000000000000, 0.000000000000000000, 0.000000000000000000 ) ) ;
#1285=VECTOR ( 'NONE', #336, 1000.000000000000000 ) ;
#1288=CARTESIAN_POINT ( 'NONE',  ( -17.18149551509903361, 19.58805710660143973, 20.00001200000000168 ) ) ;
#1292=CIRCLE ( 'NONE', #3178, 26.00000000000000355 ) ;
#1304=AXIS2_PLACEMENT_3D ( 'NONE', #4399, #879, #1873 ) ;
#1305=CARTESIAN_POINT ( 'NONE',  ( 18.19536891688249014, 23.85222316637479523, 9.261144538644668245 ) ) ;
#1308=EDGE_CURVE ( 'NONE', #2854, #305, #4148, .T. ) ;
#1309=CARTESIAN_POINT ( 'NONE',  ( -18.19536891688249014, 23.85222316637479878, 8.735393166554770161 ) ) ;
#1311=AXIS2_PLACEMENT_3D ( 'NONE', #4515, #1234, #143 ) ;
#1312=CYLINDRICAL_SURFACE ( 'NONE', #4566, 3.999999999999998224 ) ;
#1314=ORIENTED_EDGE ( 'NONE', *, *, #23, .T. ) ;
#1317=VECTOR ( 'NONE', #913, 1000.000000000000000 ) ;
#1325=FACE_OUTER_BOUND ( 'NONE', #2294, .T. ) ;
#1327=ORIENTED_EDGE ( 'NONE', *, *, #1910, .T. ) ;
#1330=CARTESIAN_POINT ( 'NONE',  ( 21.39823644064421160, 21.02820489033393159, 13.00018275065233020 ) ) ;
#1331=DIRECTION ( 'NONE',  ( 1.000000000000000000, 0.000000000000000000, 0.000000000000000000 ) ) ;
#1333=CARTESIAN_POINT ( 'NONE',  ( 30.00000000000005684, 29.99999999999995026, 8.999999999999992895 ) ) ;
#1334=CARTESIAN_POINT ( 'NONE',  ( -20.67279826512042717, 15.85973458909326084, 20.00001200000000168 ) ) ;
#1348=CARTESIAN_POINT ( 'NONE',  ( 3.469446951953614189E-15, 30.00000000000000355, 4.999999999999992006 ) ) ;
#1351=VECTOR ( 'NONE', #3175, 1000.000000000000000 ) ;
#1353=CARTESIAN_POINT ( 'NONE',  ( 18.97463723504673538, 23.23784379901355024, 11.64206388705991557 ) ) ;
#1356=FACE_OUTER_BOUND ( 'NONE', #3043, .T. ) ;
#1359=AXIS2_PLACEMENT_3D ( 'NONE', #195, #2782, #1377 ) ;
#1360=DIRECTION ( 'NONE',  ( 0.000000000000000000, 0.000000000000000000, -1.000000000000000000 ) ) ;
#1363=CARTESIAN_POINT ( 'NONE',  ( 3.959305671612554781E-15, 30.00000000000000355, 12.99999999999999289 ) ) ;
#1375=VERTEX_POINT ( 'NONE', #3406 ) ;
#1376=ORIENTED_EDGE ( 'NONE', *, *, #4469, .T. ) ;
#1377=DIRECTION ( 'NONE',  ( 1.000000000000000000, 0.000000000000000000, 0.000000000000000000 ) ) ;
#1378=ADVANCED_FACE ( 'NONE', ( #1593 ), #174, .T. ) ;
#1381=ORIENTED_EDGE ( 'NONE', *, *, #1748, .F. ) ;
#1383=CARTESIAN_POINT ( 'NONE',  ( 20.67279826512042007, 15.85973458909327860, 20.00001200000000523 ) ) ;
#1389=CARTESIAN_POINT ( 'NONE',  ( 3.179912982098363816, 29.83135056253849626, 11.44055532734088665 ) ) ;
#1393=CARTESIAN_POINT ( 'NONE',  ( -6.741346781237202102, -25.16843286583315731, 20.00001200000000168 ) ) ;
#1394=DIRECTION ( 'NONE',  ( 0.000000000000000000, 0.000000000000000000, 1.000000000000000000 ) ) ;
#1395=CARTESIAN_POINT ( 'NONE',  ( 0.000000000000000000, 10.00000000000000000, 15.00000000000000178 ) ) ;
#1403=DIRECTION ( 'NONE',  ( 1.000000000000000000, 0.000000000000000000, 0.000000000000000000 ) ) ;
#1404=EDGE_CURVE ( 'NONE', #1997, #1098, #2874, .T. ) ;
#1405=ORIENTED_EDGE ( 'NONE', *, *, #3553, .F. ) ;
#1406=DIRECTION ( 'NONE',  ( 0.000000000000000000, -0.000000000000000000, 1.000000000000000000 ) ) ;
#1407=PLANE ( 'NONE',  #902 ) ;
#1408=SHAPE_REPRESENTATION ( 'casing', ( #2928 ), #656 ) ;
#1409=CARTESIAN_POINT ( 'NONE',  ( -18.19536891688249014, 23.85222316637480233, 8.999999999999992895 ) ) ;
#1414=FACE_BOUND ( 'NONE', #1684, .T. ) ;
#1417=ADVANCED_FACE ( 'NONE', ( #2830 ), #3975, .F. ) ;
#1418=CARTESIAN_POINT ( 'NONE',  ( -22.86845070612092456, 19.41857644225268942, 5.819272910265529397 ) ) ;
#1424=PRESENTATION_STYLE_ASSIGNMENT (( #3231 ) ) ;
#1427=CARTESIAN_POINT ( 'NONE',  ( 23.36965697125207342, 11.52193136556788211, 20.00001200000000523 ) ) ;
#1429=CARTESIAN_POINT ( 'NONE',  ( 17.67766952966372429, 17.67766952966365679, 8.999999999999992895 ) ) ;
#1435=EDGE_CURVE ( 'NONE', #3477, #3682, #15, .T. ) ;
#1436=CARTESIAN_POINT ( 'NONE',  ( 18.29840776695833071, 23.77332420219740072, 7.960232512805602845 ) ) ;
#1439=CARTESIAN_POINT ( 'NONE',  ( -8.000000000000000000, 10.00000000000000178, 15.00000000000000178 ) ) ;
#1446=DIRECTION ( 'NONE',  ( 0.000000000000000000, 0.000000000000000000, 1.000000000000000000 ) ) ;
#1448=EDGE_LOOP ( 'NONE', ( #2971, #1183 ) ) ;
#1455=VECTOR ( 'NONE', #3969, 1000.000000000000000 ) ;
#1458=CARTESIAN_POINT ( 'NONE',  ( 20.83941891177998684, 21.58204166899915322, 5.025993266704736229 ) ) ;
#1461=ORIENTED_EDGE ( 'NONE', *, *, #407, .T. ) ;
#1466=VERTEX_POINT ( 'NONE', #4330 ) ;
#1471=CARTESIAN_POINT ( 'NONE',  ( -23.23784379901361419, 18.97463723504665367, 11.64206388705991557 ) ) ;
#1477=COLOUR_RGB ( '',0.8941176470588234615, 0.8941176470588234615, 0.8941176470588234615 ) ;
#1482=CARTESIAN_POINT ( 'NONE',  ( 18.51843501006192483, 23.60249532755118551, 7.226626843687536272 ) ) ;
#1483=DIRECTION ( 'NONE',  ( 0.000000000000000000, 0.000000000000000000, 1.000000000000000000 ) ) ;
#1494=CARTESIAN_POINT ( 'NONE',  ( -20.47065640071377501, 21.93211642885832191, 12.87299606428841159 ) ) ;
#1495=ADVANCED_FACE ( 'NONE', ( #262 ), #1093, .T. ) ;
#1496=CARTESIAN_POINT ( 'NONE',  ( -26.00000000000000355, 0.000000000000000000, 19.59999999999999787 ) ) ;
#1503=CARTESIAN_POINT ( 'NONE',  ( 0.000000000000000000, 0.000000000000000000, 15.00000000000000178 ) ) ;
#1504=DIRECTION ( 'NONE',  ( 1.000000000000000000, 0.000000000000000000, 0.000000000000000000 ) ) ;
#1506=DIRECTION ( 'NONE',  ( -0.000000000000000000, -0.000000000000000000, -1.000000000000000000 ) ) ;
#1512=FACE_OUTER_BOUND ( 'NONE', #2383, .T. ) ;
#1513=VERTEX_POINT ( 'NONE', #2580 ) ;
#1514=EDGE_LOOP ( 'NONE', ( #2227, #2318, #2635, #3413 ) ) ;
#1517=EDGE_CURVE ( 'NONE', #2090, #2680, #1682, .T. ) ;
#1519=CARTESIAN_POINT ( 'NONE',  ( -18.29899638405149886, 23.77287215665554143, 10.04298872102888751 ) ) ;
#1520=EDGE_CURVE ( 'NONE', #2903, #3494, #4336, .T. ) ;
#1523=ORIENTED_EDGE ( 'NONE', *, *, #227, .F. ) ;
#1528=CARTESIAN_POINT ( 'NONE',  ( -27.10000000000000497, -0.5999999999999998668, 19.59999999999999787 ) ) ;
#1530=B_SPLINE_CURVE_WITH_KNOTS ( 'NONE', 3,
 ( #321, #3686, #4386, #33, #2232, #3309, #1128, #2129, #1832, #1152, #2474, #2931, #4408, #2590, #1393, #2426, #2566, #2082, #2451, #4031, #3551, #3333, #1016, #771, #2207, #1042, #3916, #1724, #1857, #4254, #3665, #300, #1747, #3198 ),
 .UNSPECIFIED., .F., .F.,
 ( 4, 2, 2, 2, 2, 2, 2, 2, 2, 2, 2, 2, 2, 2, 2, 2, 4 ),
 ( 0.5000000000000000000, 0.5312500000000000000, 0.5625000000000000000, 0.5937500000000000000, 0.6250000000000000000, 0.6562500000000000000, 0.6875000000000000000, 0.7187500000000000000, 0.7500000000000000000, 0.7812500000000000000, 0.8125000000000000000, 0.8437500000000000000, 0.8750000000000000000, 0.9062500000000000000, 0.9375000000000000000, 0.9687500000000000000, 1.000000000000000000 ),
 .UNSPECIFIED. ) ;
#1535=ORIENTED_EDGE ( 'NONE', *, *, #2027, .T. ) ;
#1545=UNCERTAINTY_MEASURE_WITH_UNIT (LENGTH_MEASURE( 1.000000000000000082E-05 ), #651, 'distance_accuracy_value', 'NONE');
#1549=DIRECTION ( 'NONE',  ( 0.000000000000000000, 1.000000000000000000, 0.000000000000000000 ) ) ;
#1562=CARTESIAN_POINT ( 'NONE',  ( 0.000000000000000000, 0.000000000000000000, 15.00000000000000178 ) ) ;
#1569=EDGE_LOOP ( 'NONE', ( #194, #965, #2792, #1274 ) ) ;
#1572=DIRECTION ( 'NONE',  ( 0.000000000000000000, 0.000000000000000000, 1.000000000000000000 ) ) ;
#1573=CARTESIAN_POINT ( 'NONE',  ( -22.58509718322855164, 19.74742367678131316, 12.47015313278852666 ) ) ;
#1575=FACE_OUTER_BOUND ( 'NONE', #2932, .T. ) ;
#1576=EDGE_LOOP ( 'NONE', ( #4394, #4173 ) ) ;
#1577=CARTESIAN_POINT ( 'NONE',  ( 24.00000000000000355, 0.000000000000000000, 17.00000000000000000 ) ) ;
#1583=ADVANCED_FACE ( 'NONE', ( #2674 ), #4204, .T. ) ;
#1584=CARTESIAN_POINT ( 'NONE',  ( -18.19536891688249014, 23.85222316637480233, 8.999999999999992895 ) ) ;
#1586=EDGE_CURVE ( 'NONE', #2135, #289, #1654, .T. ) ;
#1589=ORIENTED_EDGE ( 'NONE', *, *, #1874, .F. ) ;
#1593=FACE_OUTER_BOUND ( 'NONE', #417, .T. ) ;
#1600=EDGE_CURVE ( 'NONE', #3514, #4523, #2273, .T. ) ;
#1601=DIRECTION ( 'NONE',  ( 0.000000000000000000, 0.000000000000000000, -1.000000000000000000 ) ) ;
#1604=CARTESIAN_POINT ( 'NONE',  ( -3.794751686895379894, 29.75919970560060079, 7.708599238039753665 ) ) ;
#1605=CARTESIAN_POINT ( 'NONE',  ( 0.000000000000000000, 10.00000000000000000, 17.00000000000000000 ) ) ;
#1613=ORIENTED_EDGE ( 'NONE', *, *, #3132, .F. ) ;
#1617=ADVANCED_FACE ( 'NONE', ( #3851 ), #164, .T. ) ;
#1618=CARTESIAN_POINT ( 'NONE',  ( 0.000000000000000000, 0.000000000000000000, 19.59999999999999787 ) ) ;
#1622=LINE ( 'NONE', #2664, #247 ) ;
#1633=CARTESIAN_POINT ( 'NONE',  ( -23.36965697125209473, 11.52193136556784481, 20.00001200000000168 ) ) ;
#1640=LINE ( 'NONE', #4503, #161 ) ;
#1645=AXIS2_PLACEMENT_3D ( 'NONE', #4289, #353, #740 ) ;
#1649=FACE_OUTER_BOUND ( 'NONE', #3543, .T. ) ;
#1652=CARTESIAN_POINT ( 'NONE',  ( 18.61605759292315199, 23.52581488222641326, 11.00403192580902711 ) ) ;
#1654=LINE ( 'NONE', #4538, #2056 ) ;
#1655=AXIS2_PLACEMENT_3D ( 'NONE', #4621, #2387, #2828 ) ;
#1657=DIRECTION ( 'NONE',  ( 0.000000000000000000, 0.000000000000000000, 1.000000000000000000 ) ) ;
#1661=EDGE_CURVE ( 'NONE', #907, #2288, #705, .T. ) ;
#1682=CIRCLE ( 'NONE', #2430, 24.00000000000000355 ) ;
#1683=CARTESIAN_POINT ( 'NONE',  ( -11.52193136556785369, 23.36965697125208052, 20.00001200000000168 ) ) ;
#1684=EDGE_LOOP ( 'NONE', ( #501, #1523 ) ) ;
#1686=ORIENTED_EDGE ( 'NONE', *, *, #3741, .T. ) ;
#1687=DIRECTION ( 'NONE',  ( 0.000000000000000000, 0.000000000000000000, 1.000000000000000000 ) ) ;
#1691=DIRECTION ( 'NONE',  ( 1.000000000000000000, 0.000000000000000000, -0.000000000000000000 ) ) ;
#1692=DIRECTION ( 'NONE',  ( -0.000000000000000000, -0.000000000000000000, 1.000000000000000000 ) ) ;
#1698=CARTESIAN_POINT ( 'NONE',  ( 22.10492369241847044, 20.28376480839707341, 12.79609622574099070 ) ) ;
#1700=EDGE_CURVE ( 'NONE', #3253, #906, #4464, .T. ) ;
#1704=CARTESIAN_POINT ( 'NONE',  ( -27.99999999999999645, 0.000000000000000000, 20.00000000000000000 ) ) ;
#1710=CARTESIAN_POINT ( 'NONE',  ( 0.000000000000000000, 10.00000000000000000, 13.00000000000000178 ) ) ;
#1712=DIRECTION ( 'NONE',  ( 0.000000000000000000, 0.000000000000000000, 1.000000000000000000 ) ) ;
#1714=CARTESIAN_POINT ( 'NONE',  ( 25.16843286583313599, 6.741346781237259833, 20.00001200000000523 ) ) ;
#1716=CARTESIAN_POINT ( 'NONE',  ( -27.10000000000000497, -0.5999999999999998668, 19.59999999999999787 ) ) ;
#1719=ORIENTED_EDGE ( 'NONE', *, *, #4105, .T. ) ;
#1720=CIRCLE ( 'NONE', #1645, 30.00000000000000355 ) ;
#1722=CARTESIAN_POINT ( 'NONE',  ( 23.77287215665559827, 18.29899638405141715, 10.04298872102887863 ) ) ;
#1724=CARTESIAN_POINT ( 'NONE',  ( 22.56362157461194329, -13.02991752792603819, 20.00001200000000523 ) ) ;
#1729=ORIENTED_EDGE ( 'NONE', *, *, #4212, .F. ) ;
#1734=B_SPLINE_CURVE_WITH_KNOTS ( 'NONE', 3,
 ( #3684, #107, #31, #431, #2186, #1908, #2999, #3285, #1471, #840, #2278, #1573, #3329, #4381, #4429, #2563, #814, #4125, #3307, #1494, #3734, #4029, #1151, #2256, #1854, #2205, #769, #480, #2930, #3663, #1519, #4077, #81, #1932 ),
 .UNSPECIFIED., .F., .F.,
 ( 4, 2, 2, 2, 2, 2, 2, 2, 2, 2, 2, 2, 2, 2, 2, 2, 4 ),
 ( 0.01251975318912558130, 0.01330204881184919238, 0.01408434443457280347, 0.01486664005729641282, 0.01564893568002002217, 0.01643123130274363325, 0.01721352692546724433, 0.01799582254819085542, 0.01877811817091446650, 0.01956041379363807758, 0.02034270941636168867, 0.02112500503908529975, 0.02190730066180891084, 0.02268959628453252192, 0.02347189190725612953, 0.02425418752997974062, 0.02503648315270335170 ),
 .UNSPECIFIED. ) ;
#1742=CARTESIAN_POINT ( 'NONE',  ( 2.642082718872652780, 29.88400461830718058, 12.01452573847769045 ) ) ;
#1744=EDGE_CURVE ( 'NONE', #3472, #1957, #2503, .T. ) ;
#1745=CARTESIAN_POINT ( 'NONE',  ( 23.23549755865092337, 18.97751144565066994, 11.64625228532890411 ) ) ;
#1747=CARTESIAN_POINT ( 'NONE',  ( 26.00000000000000711, -1.701696020694468015, 20.00001200000000168 ) ) ;
#1748=EDGE_CURVE ( 'NONE', #1466, #2542, #2354, .T. ) ;
#1751=CARTESIAN_POINT ( 'NONE',  ( -23.77332420219745757, 18.29840776695824900, 7.960232512805597516 ) ) ;
#1763=FACE_OUTER_BOUND ( 'NONE', #3403, .T. ) ;
#1771=CARTESIAN_POINT ( 'NONE',  ( -23.34254382248203541, 18.84534098761070453, 6.559627254860783019 ) ) ;
#1779=AXIS2_PLACEMENT_3D ( 'NONE', #38, #1915, #796 ) ;
#1780=CARTESIAN_POINT ( 'NONE',  ( 0.000000000000000000, 0.000000000000000000, 0.000000000000000000 ) ) ;
#1781=CARTESIAN_POINT ( 'NONE',  ( -8.000000000000000000, 10.00000000000000178, 17.00000000000000000 ) ) ;
#1782=EDGE_LOOP ( 'NONE', ( #3974, #4228 ) ) ;
#1783=DIRECTION ( 'NONE',  ( 0.000000000000000000, 0.000000000000000000, 1.000000000000000000 ) ) ;
#1785=FACE_OUTER_BOUND ( 'NONE', #1782, .T. ) ;
#1787=DIRECTION ( 'NONE',  ( 0.000000000000000000, -1.000000000000000000, 0.000000000000000000 ) ) ;
#1789=CARTESIAN_POINT ( 'NONE',  ( -25.99307600111999150, -0.5999999999999996447, 19.59999999999999787 ) ) ;
#1793=CARTESIAN_POINT ( 'NONE',  ( 0.000000000000000000, 0.000000000000000000, 20.00000000000000000 ) ) ;
#1795=CARTESIAN_POINT ( 'NONE',  ( 19.26328748721759609, 22.99914926278827210, 5.984828968106582714 ) ) ;
#1799=ORIENTED_EDGE ( 'NONE', *, *, #1073, .T. ) ;
#1802=LINE ( 'NONE', #674, #735 ) ;
#1804=EDGE_CURVE ( 'NONE', #1098, #2111, #2453, .T. ) ;
#1827=ORIENTED_EDGE ( 'NONE', *, *, #974, .T. ) ;
#1831=FACE_OUTER_BOUND ( 'NONE', #3075, .T. ) ;
#1832=CARTESIAN_POINT ( 'NONE',  ( -19.58805710660146104, -17.18149551509901940, 20.00001200000000168 ) ) ;
#1834=VECTOR ( 'NONE', #3795, 1000.000000000000000 ) ;
#1843=ORIENTED_EDGE ( 'NONE', *, *, #2029, .F. ) ;
#1844=ORIENTED_EDGE ( 'NONE', *, *, #3834, .T. ) ;
#1848=CARTESIAN_POINT ( 'NONE',  ( 27.99999999999999645, 3.429011037612588881E-15, 20.00000000000000000 ) ) ;
#1849=ORIENTED_EDGE ( 'NONE', *, *, #761, .T. ) ;
#1852=ORIENTED_EDGE ( 'NONE', *, *, #24, .T. ) ;
#1854=CARTESIAN_POINT ( 'NONE',  ( -19.26288713789795537, 22.99946665860929684, 12.01444203287435819 ) ) ;
#1855=VECTOR ( 'NONE', #1601, 1000.000000000000000 ) ;
#1857=CARTESIAN_POINT ( 'NONE',  ( 23.36965697125208408, -11.52193136556784658, 20.00001200000000168 ) ) ;
#1858=ORIENTED_EDGE ( 'NONE', *, *, #227, .T. ) ;
#1864=CARTESIAN_POINT ( 'NONE',  ( -3.471149744654747238, 29.79887180468049479, 6.994934987683496530 ) ) ;
#1872=CARTESIAN_POINT ( 'NONE',  ( 0.000000000000000000, 0.000000000000000000, 19.59999999999999787 ) ) ;
#1873=DIRECTION ( 'NONE',  ( 0.000000000000000000, 0.000000000000000000, -1.000000000000000000 ) ) ;
#1874=EDGE_CURVE ( 'NONE', #3472, #3706, #2432, .T. ) ;
#1876=VERTEX_POINT ( 'NONE', #2574 ) ;
#1878=ADVANCED_FACE ( 'NONE', ( #1179 ), #732, .F. ) ;
#1879=UNCERTAINTY_MEASURE_WITH_UNIT (LENGTH_MEASURE( 1.000000000000000082E-05 ), #2838, 'distance_accuracy_value', 'NONE');
#1881=CARTESIAN_POINT ( 'NONE',  ( -27.10000000000000497, 0.6000000000000000888, 19.59999999999999787 ) ) ;
#1883=FACE_OUTER_BOUND ( 'NONE', #4047, .T. ) ;
#1884=AXIS2_PLACEMENT_3D ( 'NONE', #2691, #4156, #2324 ) ;
#1888=DIRECTION ( 'NONE',  ( 0.000000000000000000, 0.000000000000000000, -1.000000000000000000 ) ) ;
#1890=CARTESIAN_POINT ( 'NONE',  ( 22.58414294016076695, 19.74853269256671240, 5.528858171306252345 ) ) ;
#1891=DIRECTION ( 'NONE',  ( -0.000000000000000000, -0.000000000000000000, 1.000000000000000000 ) ) ;
#1901=CARTESIAN_POINT ( 'NONE',  ( -27.10000000000000497, 0.6000000000000000888, 19.00000000000000000 ) ) ;
#1908=CARTESIAN_POINT ( 'NONE',  ( -23.60309964903850499, 18.51766120599529231, 10.77116693461329255 ) ) ;
#1910=EDGE_CURVE ( 'NONE', #1928, #3361, #1228, .T. ) ;
#1915=DIRECTION ( 'NONE',  ( 0.000000000000000000, 0.000000000000000000, 1.000000000000000000 ) ) ;
#1921=CARTESIAN_POINT ( 'NONE',  ( -26.00000000000000355, 0.000000000000000000, 20.00001200000000168 ) ) ;
#1924=DIRECTION ( 'NONE',  ( 1.000000000000000000, 0.000000000000000000, 0.000000000000000000 ) ) ;
#1928=VERTEX_POINT ( 'NONE', #2263 ) ;
#1929=EDGE_LOOP ( 'NONE', ( #2443, #882 ) ) ;
#1932=CARTESIAN_POINT ( 'NONE',  ( -18.19536891688249014, 23.85222316637480233, 8.999999999999992895 ) ) ;
#1955=EDGE_LOOP ( 'NONE', ( #1613, #2019, #1843, #401, #2113 ) ) ;
#1956=ORIENTED_EDGE ( 'NONE', *, *, #2377, .T. ) ;
#1957=VERTEX_POINT ( 'NONE', #1197 ) ;
#1959=CYLINDRICAL_SURFACE ( 'NONE', #4247, 3.999999999999998224 ) ;
#1969=CARTESIAN_POINT ( 'NONE',  ( 18.84548434425194685, 23.34243530581957771, 11.44084376890924304 ) ) ;
#1977=ORIENTED_EDGE ( 'NONE', *, *, #1034, .T. ) ;
#1978=ORIENTED_EDGE ( 'NONE', *, *, #1874, .T. ) ;
#1983=AXIS2_PLACEMENT_3D ( 'NONE', #4547, #220, #2049 ) ;
#1989=CARTESIAN_POINT ( 'NONE',  ( -1.289143957944685281, 29.97326948525437729, 12.79562863665509553 ) ) ;
#1992=CARTESIAN_POINT ( 'NONE',  ( -18.21624787168416759, 23.83633674995671470, 8.475268202211100999 ) ) ;
#1994=CARTESIAN_POINT ( 'NONE',  ( 0.000000000000000000, 0.000000000000000000, 20.00001200000000168 ) ) ;
#1997=VERTEX_POINT ( 'NONE', #1881 ) ;
#2002=EDGE_CURVE ( 'NONE', #906, #3253, #1734, .T. ) ;
#2005=ORIENTED_EDGE ( 'NONE', *, *, #611, .T. ) ;
#2009=ORIENTED_EDGE ( 'NONE', *, *, #3700, .T. ) ;
#2011=CARTESIAN_POINT ( 'NONE',  ( 19.92007681871562497, 22.43321928693944400, 12.59316242105108685 ) ) ;
#2012=LINE ( 'NONE', #3111, #4461 ) ;
#2013=CIRCLE ( 'NONE', #729, 0.7500000000000001110 ) ;
#2014=DIRECTION ( 'NONE',  ( -0.000000000000000000, -0.000000000000000000, 1.000000000000000000 ) ) ;
#2018=ORIENTED_EDGE ( 'NONE', *, *, #2084, .F. ) ;
#2019=ORIENTED_EDGE ( 'NONE', *, *, #897, .F. ) ;
#2025=DIRECTION ( 'NONE',  ( -1.000000000000000000, -0.000000000000000000, -0.000000000000000000 ) ) ;
#2026=CIRCLE ( 'NONE', #3850, 0.7500000000000001110 ) ;
#2027=EDGE_CURVE ( 'NONE', #2482, #181, #57, .T. ) ;
#2029=EDGE_CURVE ( 'NONE', #2036, #1997, #3100, .T. ) ;
#2030=VERTEX_POINT ( 'NONE', #1224 ) ;
#2036=VERTEX_POINT ( 'NONE', #817 ) ;
#2037=CARTESIAN_POINT ( 'NONE',  ( -2.642157743709451889, 29.88401080970086099, 12.01472878375391140 ) ) ;
#2038=CARTESIAN_POINT ( 'NONE',  ( 27.09999999999999787, 0.6000000000000000888, 19.59999999999999787 ) ) ;
#2039=CIRCLE ( 'NONE', #4093, 24.00000000000000355 ) ;
#2040=CARTESIAN_POINT ( 'NONE',  ( -21.93550942649232383, 20.46703030200853135, 5.128274502689557757 ) ) ;
#2043=DIRECTION ( 'NONE',  ( 0.000000000000000000, 0.000000000000000000, 1.000000000000000000 ) ) ;
#2049=DIRECTION ( 'NONE',  ( -1.000000000000000000, 0.000000000000000000, 0.000000000000000000 ) ) ;
#2050=CARTESIAN_POINT ( 'NONE',  ( 0.000000000000000000, 10.00000000000000000, 13.00000000000000178 ) ) ;
#2056=VECTOR ( 'NONE', #2014, 1000.000000000000000 ) ;
#2065=CARTESIAN_POINT ( 'NONE',  ( -25.83240171513484640, 3.403349963601426165, 20.00001199999999812 ) ) ;
#2067=ORIENTED_EDGE ( 'NONE', *, *, #3106, .T. ) ;
#2073=CARTESIAN_POINT ( 'NONE',  ( 6.741346781237198549, 25.16843286583315020, 20.00001200000000168 ) ) ;
#2078=EDGE_CURVE ( 'NONE', #3924, #127, #3028, .T. ) ;
#2081=VECTOR ( 'NONE', #3154, 1000.000000000000000 ) ;
#2082=CARTESIAN_POINT ( 'NONE',  ( 1.701696020694480449, -26.00000000000000355, 20.00001200000000878 ) ) ;
#2084=EDGE_CURVE ( 'NONE', #1876, #2731, #3077, .T. ) ;
#2085=VECTOR ( 'NONE', #3079, 1000.000000000000000 ) ;
#2090=VERTEX_POINT ( 'NONE', #1577 ) ;
#2100=CARTESIAN_POINT ( 'NONE',  ( 3.470161297262016831, 29.79898158544631670, 11.00652372288853975 ) ) ;
#2104=CARTESIAN_POINT ( 'NONE',  ( 23.60157000768436930, 18.51961241432701399, 10.77614164618340631 ) ) ;
#2106=CARTESIAN_POINT ( 'NONE',  ( -22.43020886076084253, 19.92346879083515176, 5.404597446377701786 ) ) ;
#2111=VERTEX_POINT ( 'NONE', #157 ) ;
#2113=ORIENTED_EDGE ( 'NONE', *, *, #1035, .F. ) ;
#2116=DIRECTION ( 'NONE',  ( -0.000000000000000000, -0.000000000000000000, -1.000000000000000000 ) ) ;
#2118=CIRCLE ( 'NONE', #1135, 30.00000000000000355 ) ;
#2121=CARTESIAN_POINT ( 'NONE',  ( 30.00000000000000355, 3.673940397442059967E-15, 0.000000000000000000 ) ) ;
#2125=CARTESIAN_POINT ( 'NONE',  ( 0.5260335297454653558, 29.99650222249029952, 5.025987840185457856 ) ) ;
#2129=CARTESIAN_POINT ( 'NONE',  ( -20.67279826512042007, -15.85973458909327150, 20.00001200000000168 ) ) ;
#2135=VERTEX_POINT ( 'NONE', #3005 ) ;
#2139=EDGE_CURVE ( 'NONE', #1375, #4484, #176, .T. ) ;
#2141=CARTESIAN_POINT ( 'NONE',  ( 26.00000000000000711, 1.701696020694481559, 20.00001200000000523 ) ) ;
#2147=CARTESIAN_POINT ( 'NONE',  ( 2.440861994934926837, 29.90134041232742490, 12.17981090101949349 ) ) ;
#2158=CARTESIAN_POINT ( 'NONE',  ( 0.000000000000000000, 0.000000000000000000, 19.00000000000000000 ) ) ;
#2162=ORIENTED_EDGE ( 'NONE', *, *, #749, .T. ) ;
#2163=CARTESIAN_POINT ( 'NONE',  ( -1.701696020694479783, 25.99999999999999645, 20.00001200000000523 ) ) ;
#2164=AXIS2_PLACEMENT_3D ( 'NONE', #4030, #770, #2206 ) ;
#2165=DIRECTION ( 'NONE',  ( 0.7071067811865487940, 0.7071067811865463515, -0.000000000000000000 ) ) ;
#2169=AXIS2_PLACEMENT_3D ( 'NONE', #1994, #2802, #3808 ) ;
#2184=AXIS2_PLACEMENT_3D ( 'NONE', #1429, #2165, #3237 ) ;
#2186=CARTESIAN_POINT ( 'NONE',  ( -23.72657184721640533, 18.35919055844626158, 10.28976100101469981 ) ) ;
#2194=CARTESIAN_POINT ( 'NONE',  ( -25.99307600111999150, -0.5999999999999998668, 20.00001200000000168 ) ) ;
#2198=ORIENTED_EDGE ( 'NONE', *, *, #3857, .T. ) ;
#2199=DIRECTION ( 'NONE',  ( 0.000000000000000000, 0.000000000000000000, 1.000000000000000000 ) ) ;
#2200=LINE ( 'NONE', #1848, #698 ) ;
#2205=CARTESIAN_POINT ( 'NONE',  ( -18.97751144565075165, 23.23549755865085231, 11.64625228532891121 ) ) ;
#2206=DIRECTION ( 'NONE',  ( -1.000000000000000000, 0.000000000000000000, 0.000000000000000000 ) ) ;
#2207=CARTESIAN_POINT ( 'NONE',  ( 17.18149551509901585, -19.58805710660145749, 20.00001200000000168 ) ) ;
#2212=PLANE ( 'NONE',  #3222 ) ;
#2215=CARTESIAN_POINT ( 'NONE',  ( 23.52555220673924197, 18.61638332444494992, 6.995423750305945987 ) ) ;
#2216=CARTESIAN_POINT ( 'NONE',  ( -3.178742173564956808, 29.83148068024111410, 6.557713274934318548 ) ) ;
#2220=ORIENTED_EDGE ( 'NONE', *, *, #2538, .F. ) ;
#2227=ORIENTED_EDGE ( 'NONE', *, *, #1700, .T. ) ;
#2232=CARTESIAN_POINT ( 'NONE',  ( -24.67207871933483432, -8.377607117416806304, 20.00001200000000168 ) ) ;
#2233=ORIENTED_EDGE ( 'NONE', *, *, #4105, .F. ) ;
#2236=EDGE_CURVE ( 'NONE', #906, #3494, #3124, .T. ) ;
#2240=DIRECTION ( 'NONE',  ( 1.000000000000000000, 0.000000000000000000, 0.000000000000000000 ) ) ;
#2245=EDGE_LOOP ( 'NONE', ( #533, #394, #151, #3056 ) ) ;
#2246=DIRECTION ( 'NONE',  ( 0.000000000000000000, 0.000000000000000000, -1.000000000000000000 ) ) ;
#2250=ORIENTED_EDGE ( 'NONE', *, *, #363, .T. ) ;
#2256=CARTESIAN_POINT ( 'NONE',  ( -19.42075468095228530, 22.86660962422639898, 12.18297904795690378 ) ) ;
#2263=CARTESIAN_POINT ( 'NONE',  ( 23.85222316637486273, 18.19536891688240843, 8.999999999999992895 ) ) ;
#2264=CARTESIAN_POINT ( 'NONE',  ( -2.439210544738880326, 29.90146712018378494, 5.819033386899011617 ) ) ;
#2266=ORIENTED_EDGE ( 'NONE', *, *, #4287, .F. ) ;
#2273=CIRCLE ( 'NONE', #4123, 0.7500000000000001110 ) ;
#2278=CARTESIAN_POINT ( 'NONE',  ( -22.86919556969945333, 19.41770456673549106, 12.17989986600643348 ) ) ;
#2286=CARTESIAN_POINT ( 'NONE',  ( -0.5247320085691752345, 29.99650235037416834, 5.025996973432255821 ) ) ;
#2287=CYLINDRICAL_SURFACE ( 'NONE', #3998, 30.00000000000000355 ) ;
#2288=VERTEX_POINT ( 'NONE', #3569 ) ;
#2289=ADVANCED_FACE ( 'NONE', ( #1763 ), #1031, .F. ) ;
#2290=DIRECTION ( 'NONE',  ( 0.000000000000000000, -0.000000000000000000, 1.000000000000000000 ) ) ;
#2294=EDGE_LOOP ( 'NONE', ( #3003, #772, #1052, #3609 ) ) ;
#2300=VECTOR ( 'NONE', #1088, 1000.000000000000000 ) ;
#2304=DIRECTION ( 'NONE',  ( 1.000000000000000000, 0.000000000000000000, 0.000000000000000000 ) ) ;
#2305=DIRECTION ( 'NONE',  ( 0.000000000000000000, -1.000000000000000000, 0.000000000000000000 ) ) ;
#2308=VECTOR ( 'NONE', #1549, 1000.000000000000000 ) ;
#2312=CARTESIAN_POINT ( 'NONE',  ( -19.41638709359449422, 22.87032942663237378, 5.821272343678753458 ) ) ;
#2317=ORIENTED_EDGE ( 'NONE', *, *, #724, .F. ) ;
#2318=ORIENTED_EDGE ( 'NONE', *, *, #2236, .T. ) ;
#2319=ORIENTED_EDGE ( 'NONE', *, *, #2646, .F. ) ;
#2324=DIRECTION ( 'NONE',  ( 1.000000000000000000, 0.000000000000000000, -0.000000000000000000 ) ) ;
#2328=CARTESIAN_POINT ( 'NONE',  ( -1.773386257881301553, 29.94852044693267246, 12.59496732558994125 ) ) ;
#2334=FACE_OUTER_BOUND ( 'NONE', #105, .T. ) ;
#2335=CARTESIAN_POINT ( 'NONE',  ( -19.58805710660148236, 17.18149551509898743, 20.00001200000000523 ) ) ;
#2340=FACE_OUTER_BOUND ( 'NONE', #747, .T. ) ;
#2341=DIRECTION ( 'NONE',  ( 0.000000000000000000, 0.000000000000000000, -1.000000000000000000 ) ) ;
#2346=CARTESIAN_POINT ( 'NONE',  ( -27.10000000000000497, 0.6000000000000000888, 19.59999999999999787 ) ) ;
#2347=FACE_OUTER_BOUND ( 'NONE', #1929, .T. ) ;
#2351=CARTESIAN_POINT ( 'NONE',  ( -3.595408253811773758, 29.78394301743083261, 10.77252090037689136 ) ) ;
#2354=CIRCLE ( 'NONE', #4045, 4.000000000000000000 ) ;
#2357=DIRECTION ( 'NONE',  ( 0.000000000000000000, 0.000000000000000000, -1.000000000000000000 ) ) ;
#2362=ORIENTED_EDGE ( 'NONE', *, *, #4531, .F. ) ;
#2369=DIRECTION ( 'NONE',  ( 0.000000000000000000, 0.000000000000000000, -1.000000000000000000 ) ) ;
#2370=DIRECTION ( 'NONE',  ( 1.000000000000000000, 0.000000000000000000, 0.000000000000000000 ) ) ;
#2376=CARTESIAN_POINT ( 'NONE',  ( 20.83769629064231665, 21.58369355588040861, 12.97362800538644301 ) ) ;
#2377=EDGE_CURVE ( 'NONE', #741, #305, #1149, .T. ) ;
#2379=CIRCLE ( 'NONE', #1107, 8.000000000000000000 ) ;
#2380=CARTESIAN_POINT ( 'NONE',  ( -21.39687781493365293, 21.02954719696279895, 4.999903794384585431 ) ) ;
#2383=EDGE_LOOP ( 'NONE', ( #1849, #4478 ) ) ;
#2387=DIRECTION ( 'NONE',  ( 0.000000000000000000, 0.000000000000000000, 1.000000000000000000 ) ) ;
#2388=ADVANCED_FACE ( 'NONE', ( #1785 ), #4335, .T. ) ;
#2394=CARTESIAN_POINT ( 'NONE',  ( 0.000000000000000000, 0.000000000000000000, 19.00000000000000000 ) ) ;
#2395=EDGE_CURVE ( 'NONE', #1928, #2542, #3284, .T. ) ;
#2403=CARTESIAN_POINT ( 'NONE',  ( 25.99307600111999150, 0.5999999999999998668, 19.00000000000000000 ) ) ;
#2406=VECTOR ( 'NONE', #1360, 1000.000000000000000 ) ;
#2409=EDGE_LOOP ( 'NONE', ( #1978, #3352 ) ) ;
#2411=DIRECTION ( 'NONE',  ( 0.7071067811865487940, 0.7071067811865463515, 0.000000000000000000 ) ) ;
#2421=CARTESIAN_POINT ( 'NONE',  ( 3.999815009702282875, 29.73216238221898067, 9.267216418983164061 ) ) ;
#2425=CARTESIAN_POINT ( 'NONE',  ( -3.015186248472646824, 29.84868090056883716, 11.64163568064553544 ) ) ;
#2426=CARTESIAN_POINT ( 'NONE',  ( -3.403349963601427053, -25.83240171513484640, 20.00001199999999812 ) ) ;
#2430=AXIS2_PLACEMENT_3D ( 'NONE', #1143, #373, #830 ) ;
#2431=CYLINDRICAL_SURFACE ( 'NONE', #2169, 26.00000000000000355 ) ;
#2432=CIRCLE ( 'NONE', #318, 27.99999999999999645 ) ;
#2433=ORIENTED_EDGE ( 'NONE', *, *, #3215, .F. ) ;
#2439=CARTESIAN_POINT ( 'NONE',  ( -8.377607117416806304, 24.67207871933483787, 20.00001200000000168 ) ) ;
#2442=CARTESIAN_POINT ( 'NONE',  ( 3.014458645203628606, 29.84873923156943576, 6.357858316023347278 ) ) ;
#2443=ORIENTED_EDGE ( 'NONE', *, *, #4560, .T. ) ;
#2447=PLANE ( 'NONE',  #2684 ) ;
#2451=CARTESIAN_POINT ( 'NONE',  ( 3.403349963601436823, -25.83240171513484995, 20.00001200000000878 ) ) ;
#2453=LINE ( 'NONE', #712, #3582 ) ;
#2457=ORIENTED_EDGE ( 'NONE', *, *, #45, .F. ) ;
#2460=CARTESIAN_POINT ( 'NONE',  ( 0.000000000000000000, 0.000000000000000000, 20.00001200000000168 ) ) ;
#2474=CARTESIAN_POINT ( 'NONE',  ( -15.85973458909327150, -20.67279826512042362, 20.00001200000000168 ) ) ;
#2479=CARTESIAN_POINT ( 'NONE',  ( 0.000000000000000000, 10.00000000000000000, 15.00000000000000178 ) ) ;
#2482=VERTEX_POINT ( 'NONE', #2516 ) ;
#2490=CARTESIAN_POINT ( 'NONE',  ( -17.67766952966371719, 17.67766952966366389, 8.999999999999992895 ) ) ;
#2494=DIRECTION ( 'NONE',  ( -0.000000000000000000, -0.000000000000000000, 1.000000000000000000 ) ) ;
#2497=CARTESIAN_POINT ( 'NONE',  ( 23.85222316637486983, 18.19536891688241198, 9.264542937126584832 ) ) ;
#2500=ADVANCED_BREP_SHAPE_REPRESENTATION ( '', ( #2883, #2928 ), #656 ) ;
#2502=ADVANCED_FACE ( 'NONE', ( #1055 ), #1407, .T. ) ;
#2503=LINE ( 'NONE', #1704, #1455 ) ;
#2508=DIRECTION ( 'NONE',  ( 0.000000000000000000, 0.000000000000000000, -1.000000000000000000 ) ) ;
#2510=EDGE_CURVE ( 'NONE', #3253, #2903, #4404, .T. ) ;
#2513=CARTESIAN_POINT ( 'NONE',  ( 13.02991752792603108, 22.56362157461194329, 20.00001200000000168 ) ) ;
#2516=CARTESIAN_POINT ( 'NONE',  ( -0.5000000000000001110, 10.00000000000000000, 13.00000000000000178 ) ) ;
#2518=CARTESIAN_POINT ( 'NONE',  ( 3.182992266941310433, 29.83102156157410434, 6.563430084856013202 ) ) ;
#2520=CARTESIAN_POINT ( 'NONE',  ( 23.72542776831235400, 18.36067068532939572, 10.29518969959635477 ) ) ;
#2522=DIRECTION ( 'NONE',  ( 0.000000000000000000, 0.000000000000000000, 1.000000000000000000 ) ) ;
#2526=EDGE_LOOP ( 'NONE', ( #2018, #117, #69, #3908 ) ) ;
#2532=EDGE_LOOP ( 'NONE', ( #2656, #4200 ) ) ;
#2538=EDGE_CURVE ( 'NONE', #3361, #1466, #1170, .T. ) ;
#2541=LINE ( 'NONE', #2954, #2618 ) ;
#2542=VERTEX_POINT ( 'NONE', #1271 ) ;
#2546=CIRCLE ( 'NONE', #3168, 26.00000000000000355 ) ;
#2547=FACE_OUTER_BOUND ( 'NONE', #2409, .T. ) ;
#2549=CARTESIAN_POINT ( 'NONE',  ( 23.77384460521241394, 18.29773070266329782, 7.963596978677151661 ) ) ;
#2552=VERTEX_POINT ( 'NONE', #152 ) ;
#2556=CARTESIAN_POINT ( 'NONE',  ( 0.000000000000000000, 10.00000000000000000, 15.00000000000000178 ) ) ;
#2557=ORIENTED_EDGE ( 'NONE', *, *, #4589, .F. ) ;
#2558=ORIENTED_EDGE ( 'NONE', *, *, #283, .T. ) ;
#2560=CIRCLE ( 'NONE', #3628, 27.99999999999999645 ) ;
#2563=CARTESIAN_POINT ( 'NONE',  ( -21.58369355588047966, 20.83769629064224915, 12.97362800538644301 ) ) ;
#2565=FACE_BOUND ( 'NONE', #3933, .T. ) ;
#2566=CARTESIAN_POINT ( 'NONE',  ( -1.701696020694465128, -26.00000000000001066, 20.00001200000000878 ) ) ;
#2574=CARTESIAN_POINT ( 'NONE',  ( 27.09999999999999787, -0.5999999999999998668, 19.00000000000000000 ) ) ;
#2580=CARTESIAN_POINT ( 'NONE',  ( 8.000000000000000000, 10.00000000000000000, 17.00000000000000000 ) ) ;
#2582=CARTESIAN_POINT ( 'NONE',  ( 3.469446951953614189E-15, 25.00000000000000000, 8.999999999999992895 ) ) ;
#2584=EDGE_LOOP ( 'NONE', ( #3783, #3183 ) ) ;
#2588=CARTESIAN_POINT ( 'NONE',  ( -0.5000000000000001110, 10.00000000000000000, 13.00000000000000178 ) ) ;
#2589=DIRECTION ( 'NONE',  ( -0.000000000000000000, -0.000000000000000000, 1.000000000000000000 ) ) ;
#2590=CARTESIAN_POINT ( 'NONE',  ( -8.377607117416792093, -24.67207871933483787, 20.00001200000000168 ) ) ;
#2593=ORIENTED_EDGE ( 'NONE', *, *, #1035, .T. ) ;
#2604=ORIENTED_EDGE ( 'NONE', *, *, #4469, .F. ) ;
#2611=ORIENTED_EDGE ( 'NONE', *, *, #611, .F. ) ;
#2618=VECTOR ( 'NONE', #1104, 1000.000000000000000 ) ;
#2623=CARTESIAN_POINT ( 'NONE',  ( 19.92346879083522637, 22.43020886076077502, 5.404597446377704451 ) ) ;
#2635=ORIENTED_EDGE ( 'NONE', *, *, #1520, .F. ) ;
#2646=EDGE_CURVE ( 'NONE', #3706, #3472, #2560, .T. ) ;
#2647=DIRECTION ( 'NONE',  ( 1.000000000000000000, 0.000000000000000000, 0.000000000000000000 ) ) ;
#2648=FACE_OUTER_BOUND ( 'NONE', #351, .T. ) ;
#2653=DIRECTION ( 'NONE',  ( 0.000000000000000000, 1.000000000000000000, 0.000000000000000000 ) ) ;
#2656=ORIENTED_EDGE ( 'NONE', *, *, #3834, .F. ) ;
#2664=CARTESIAN_POINT ( 'NONE',  ( 27.09999999999999787, -0.5999999999999998668, 19.59999999999999787 ) ) ;
#2666=CARTESIAN_POINT ( 'NONE',  ( 0.000000000000000000, 10.00000000000000000, 15.00000000000000178 ) ) ;
#2669=VECTOR ( 'NONE', #4155, 1000.000000000000000 ) ;
#2671=DIRECTION ( 'NONE',  ( 1.000000000000000000, 0.000000000000000000, 0.000000000000000000 ) ) ;
#2674=FACE_OUTER_BOUND ( 'NONE', #3471, .T. ) ;
#2679=VERTEX_POINT ( 'NONE', #910 ) ;
#2680=VERTEX_POINT ( 'NONE', #3757 ) ;
#2684=AXIS2_PLACEMENT_3D ( 'NONE', #1793, #275, #730 ) ;
#2688=ADVANCED_FACE ( 'NONE', ( #2340 ), #1959, .F. ) ;
#2691=CARTESIAN_POINT ( 'NONE',  ( 0.000000000000000000, 0.000000000000000000, 15.00000000000000178 ) ) ;
#2695=( GEOMETRIC_REPRESENTATION_CONTEXT ( 3 ) GLOBAL_UNCERTAINTY_ASSIGNED_CONTEXT ( ( #1545 ) ) GLOBAL_UNIT_ASSIGNED_CONTEXT ( ( #651, #4625, #2808 ) ) REPRESENTATION_CONTEXT ( 'NONE', 'WORKASPACE' ) );
#2696=CARTESIAN_POINT ( 'NONE',  ( 0.7500000000000001110, 0.000000000000000000, 15.00000000000000178 ) ) ;
#2699=VECTOR ( 'NONE', #644, 1000.000000000000000 ) ;
#2700=CARTESIAN_POINT ( 'NONE',  ( -19.92335677698585172, 22.43029000766435388, 5.404794703904383546 ) ) ;
#2701=DIRECTION ( 'NONE',  ( 0.7071067811865462405, -0.7071067811865487940, 0.000000000000000000 ) ) ;
#2704=AXIS2_PLACEMENT_3D ( 'NONE', #4664, #2843, #4079 ) ;
#2706=ORIENTED_EDGE ( 'NONE', *, *, #3917, .T. ) ;
#2709=ORIENTED_EDGE ( 'NONE', *, *, #2002, .T. ) ;
#2713=DIRECTION ( 'NONE',  ( 1.000000000000000000, 0.000000000000000000, 0.000000000000000000 ) ) ;
#2714=DIRECTION ( 'NONE',  ( -0.000000000000000000, -0.000000000000000000, -1.000000000000000000 ) ) ;
#2719=PLANE ( 'NONE',  #340 ) ;
#2722=ADVANCED_FACE ( 'NONE', ( #3096, #3474 ), #4240, .T. ) ;
#2724=CARTESIAN_POINT ( 'NONE',  ( 20.28006516365571699, 22.10831845702701060, 12.79440425686131988 ) ) ;
#2727=DIRECTION ( 'NONE',  ( -0.000000000000000000, 1.000000000000000000, 0.000000000000000000 ) ) ;
#2730=FACE_OUTER_BOUND ( 'NONE', #3558, .T. ) ;
#2731=VERTEX_POINT ( 'NONE', #4647 ) ;
#2745=CARTESIAN_POINT ( 'NONE',  ( -3.974007292349814424, 29.73566758725665338, 9.525109153848150711 ) ) ;
#2750=ADVANCED_FACE ( 'NONE', ( #240 ), #4286, .F. ) ;
#2751=CARTESIAN_POINT ( 'NONE',  ( -18.97646788767675119, 23.23634976112692740, 6.355262957884884045 ) ) ;
#2753=CARTESIAN_POINT ( 'NONE',  ( -22.56362157461194329, 13.02991752792602931, 20.00001200000000168 ) ) ;
#2761=CARTESIAN_POINT ( 'NONE',  ( -0.7500000000000001110, 9.184850993605150903E-17, 15.00000000000000178 ) ) ;
#2765=DIRECTION ( 'NONE',  ( 0.000000000000000000, 0.000000000000000000, 1.000000000000000000 ) ) ;
#2767=B_SPLINE_CURVE_WITH_KNOTS ( 'NONE', 3,
 ( #3960, #2141, #3169, #1714, #4652, #1427, #2879, #1383, #2810, #2833, #1077, #2513, #3980, #629, #2073, #721, #3520, #2163, #242, #1005, #2439, #1683, #212, #4170, #1288, #2335, #1334, #2753, #1633, #187, #3827, #2065, #978, #569 ),
 .UNSPECIFIED., .F., .F.,
 ( 4, 2, 2, 2, 2, 2, 2, 2, 2, 2, 2, 2, 2, 2, 2, 2, 4 ),
 ( 0.000000000000000000, 0.03124999999999998612, 0.06249999999999995837, 0.09374999999999993061, 0.1249999999999999029, 0.1562499999999998890, 0.1874999999999998890, 0.2187499999999998890, 0.2499999999999998890, 0.2812499999999998890, 0.3124999999999998890, 0.3437499999999998335, 0.3749999999999998335, 0.4062499999999998335, 0.4374999999999998335, 0.4687499999999998890, 0.5000000000000000000 ),
 .UNSPECIFIED. ) ;
#2769=VECTOR ( 'NONE', #3103, 1000.000000000000000 ) ;
#2770=CARTESIAN_POINT ( 'NONE',  ( -0.2612076306139402004, 30.00000000000001066, 12.99999999999999467 ) ) ;
#2771=DIRECTION ( 'NONE',  ( 0.000000000000000000, 0.000000000000000000, 1.000000000000000000 ) ) ;
#2773=EDGE_CURVE ( 'NONE', #2542, #1466, #3107, .T. ) ;
#2779=ORIENTED_EDGE ( 'NONE', *, *, #1586, .F. ) ;
#2782=DIRECTION ( 'NONE',  ( -0.000000000000000000, -0.000000000000000000, 1.000000000000000000 ) ) ;
#2785=AXIS2_PLACEMENT_3D ( 'NONE', #2556, #1446, #1403 ) ;
#2788=LINE ( 'NONE', #1363, #3138 ) ;
#2791=CARTESIAN_POINT ( 'NONE',  ( 2.646272448955801160, 29.88363158593299929, 5.989166937914467859 ) ) ;
#2792=ORIENTED_EDGE ( 'NONE', *, *, #4212, .T. ) ;
#2796=CARTESIAN_POINT ( 'NONE',  ( -3.871726839561290490, 29.74915783848840434, 10.03836643961818886 ) ) ;
#2797=LINE ( 'NONE', #994, #1351 ) ;
#2802=DIRECTION ( 'NONE',  ( 0.000000000000000000, 0.000000000000000000, -1.000000000000000000 ) ) ;
#2808=( NAMED_UNIT ( * ) SI_UNIT ( $, .STERADIAN. ) SOLID_ANGLE_UNIT ( ) );
#2809=PRODUCT_DEFINITION_CONTEXT ( 'detailed design', #3191, 'design' ) ;
#2810=CARTESIAN_POINT ( 'NONE',  ( 19.58805710660146815, 17.18149551509899453, 20.00001200000000168 ) ) ;
#2811=EDGE_CURVE ( 'NONE', #2036, #1146, #3833, .T. ) ;
#2813=DIRECTION ( 'NONE',  ( 0.000000000000000000, 0.000000000000000000, 1.000000000000000000 ) ) ;
#2814=CARTESIAN_POINT ( 'NONE',  ( 0.2645425327012488337, 30.00000000000001066, 4.999999999999992006 ) ) ;
#2817=( NAMED_UNIT ( * ) PLANE_ANGLE_UNIT ( ) SI_UNIT ( $, .RADIAN. ) );
#2820=PLANE ( 'NONE',  #2704 ) ;
#2828=DIRECTION ( 'NONE',  ( 1.000000000000000000, 0.000000000000000000, -0.000000000000000000 ) ) ;
#2830=FACE_OUTER_BOUND ( 'NONE', #4160, .T. ) ;
#2831=DIRECTION ( 'NONE',  ( -0.000000000000000000, -0.000000000000000000, 1.000000000000000000 ) ) ;
#2833=CARTESIAN_POINT ( 'NONE',  ( 17.18149551509901940, 19.58805710660145039, 20.00001200000000168 ) ) ;
#2836=CARTESIAN_POINT ( 'NONE',  ( 3.959305739469038251E-15, 30.00000000000000355, 12.99999999999999289 ) ) ;
#2837=EDGE_CURVE ( 'NONE', #2135, #2482, #365, .T. ) ;
#2838=( LENGTH_UNIT ( ) NAMED_UNIT ( * ) SI_UNIT ( .MILLI., .METRE. ) );
#2843=DIRECTION ( 'NONE',  ( 0.000000000000000000, 0.000000000000000000, 1.000000000000000000 ) ) ;
#2854=VERTEX_POINT ( 'NONE', #648 ) ;
#2860=CARTESIAN_POINT ( 'NONE',  ( 3.974400453438903025, 29.73561427688381187, 8.478299341892736152 ) ) ;
#2864=CARTESIAN_POINT ( 'NONE',  ( 30.00000000000000355, 3.673940397442059967E-15, 17.99999999999998579 ) ) ;
#2869=CIRCLE ( 'NONE', #4545, 0.5000000000000001110 ) ;
#2872=ORIENTED_EDGE ( 'NONE', *, *, #4560, .F. ) ;
#2874=LINE ( 'NONE', #1049, #3277 ) ;
#2879=CARTESIAN_POINT ( 'NONE',  ( 22.56362157461193618, 13.02991752792604174, 20.00001200000000168 ) ) ;
#2880=CARTESIAN_POINT ( 'NONE',  ( 32.82842712474624136, 27.17157287525375509, 8.999999999999992895 ) ) ;
#2882=CARTESIAN_POINT ( 'NONE',  ( 2.008133535499844413, 29.93351678898486057, 5.530618255832751018 ) ) ;
#2883=MANIFOLD_SOLID_BREP ( 'Cut-Extrude7', #4347 ) ;
#2886=DIRECTION ( 'NONE',  ( 0.000000000000000000, 0.000000000000000000, -1.000000000000000000 ) ) ;
#2890=CARTESIAN_POINT ( 'NONE',  ( 18.21639843360786770, 23.83622240491800426, 8.473444514228560820 ) ) ;
#2903=VERTEX_POINT ( 'NONE', #591 ) ;
#2909=ORIENTED_EDGE ( 'NONE', *, *, #2084, .T. ) ;
#2911=CARTESIAN_POINT ( 'NONE',  ( 23.34033764136075817, 18.84808613845415337, 11.44520879210846154 ) ) ;
#2913=CARTESIAN_POINT ( 'NONE',  ( 19.41857644225276402, 22.86845070612086417, 5.819272910265532950 ) ) ;
#2928=AXIS2_PLACEMENT_3D ( 'NONE', #1780, #1712, #3957 ) ;
#2930=CARTESIAN_POINT ( 'NONE',  ( -18.51961241432708505, 23.60157000768430535, 10.77614164618340808 ) ) ;
#2931=CARTESIAN_POINT ( 'NONE',  ( -13.02991752792603997, -22.56362157461194684, 20.00001200000000168 ) ) ;
#2932=EDGE_LOOP ( 'NONE', ( #3351, #1719 ) ) ;
#2934=VECTOR ( 'NONE', #3367, 1000.000000000000000 ) ;
#2937=CARTESIAN_POINT ( 'NONE',  ( 8.000000000000000000, 10.00000000000000000, 15.00000000000000178 ) ) ;
#2940=CARTESIAN_POINT ( 'NONE',  ( 23.00034469605617815, 19.26183863435811006, 5.986743120287543185 ) ) ;
#2942=CARTESIAN_POINT ( 'NONE',  ( 0.000000000000000000, 0.000000000000000000, 20.00000000000000000 ) ) ;
#2949=ORIENTED_EDGE ( 'NONE', *, *, #171, .T. ) ;
#2954=CARTESIAN_POINT ( 'NONE',  ( -30.00000000000000355, 0.000000000000000000, 20.00000000000000000 ) ) ;
#2961=DIRECTION ( 'NONE',  ( -1.000000000000000000, 0.000000000000000000, 0.000000000000000000 ) ) ;
#2962=CARTESIAN_POINT ( 'NONE',  ( 21.39894891851820091, 21.02743970908333182, 5.000096751259998307 ) ) ;
#2969=VERTEX_POINT ( 'NONE', #4033 ) ;
#2971=ORIENTED_EDGE ( 'NONE', *, *, #1520, .T. ) ;
#2975=CYLINDRICAL_SURFACE ( 'NONE', #268, 8.000000000000000000 ) ;
#2985=CARTESIAN_POINT ( 'NONE',  ( 21.93593546006599126, 20.46659425767087015, 5.128325996195414405 ) ) ;
#2986=DIRECTION ( 'NONE',  ( 0.000000000000000000, 0.000000000000000000, -1.000000000000000000 ) ) ;
#2995=VERTEX_POINT ( 'NONE', #1789 ) ;
#2999=CARTESIAN_POINT ( 'NONE',  ( -23.52581488222647010, 18.61605759292307383, 11.00403192580902711 ) ) ;
#3003=ORIENTED_EDGE ( 'NONE', *, *, #2029, .T. ) ;
#3005=CARTESIAN_POINT ( 'NONE',  ( 0.5000000000000001110, 10.00000000000000000, 13.00000000000000178 ) ) ;
#3009=AXIS2_PLACEMENT_3D ( 'NONE', #3824, #1282, #2771 ) ;
#3023=DIRECTION ( 'NONE',  ( 1.000000000000000000, 0.000000000000000000, 0.000000000000000000 ) ) ;
#3025=PLANE ( 'NONE',  #4686 ) ;
#3028=LINE ( 'NONE', #3362, #707 ) ;
#3038=DIRECTION ( 'NONE',  ( 0.000000000000000000, -0.000000000000000000, 1.000000000000000000 ) ) ;
#3043=EDGE_LOOP ( 'NONE', ( #3064, #1858, #2005, #3839, #3189, #1193, #1956, #1162 ) ) ;
#3044=ADVANCED_FACE ( 'NONE', ( #893, #2347 ), #535, .T. ) ;
#3049=DIRECTION ( 'NONE',  ( 0.000000000000000000, 0.000000000000000000, 1.000000000000000000 ) ) ;
#3051=PRODUCT_DEFINITION_SHAPE ( 'NONE', 'NONE',  #3648 ) ;
#3053=CARTESIAN_POINT ( 'NONE',  ( 3.469446951953614189E-15, 25.00000000000000000, 8.999999999999992895 ) ) ;
#3054=CARTESIAN_POINT ( 'NONE',  ( 25.99307600111999150, -0.5999999999999996447, 19.59999999999999787 ) ) ;
#3056=ORIENTED_EDGE ( 'NONE', *, *, #1661, .T. ) ;
#3057=AXIS2_PLACEMENT_3D ( 'NONE', #224, #4628, #988 ) ;
#3059=DIRECTION ( 'NONE',  ( 0.000000000000000000, 0.000000000000000000, -1.000000000000000000 ) ) ;
#3064=ORIENTED_EDGE ( 'NONE', *, *, #1260, .F. ) ;
#3068=ORIENTED_EDGE ( 'NONE', *, *, #3215, .T. ) ;
#3069=CARTESIAN_POINT ( 'NONE',  ( 30.00000000000005684, 29.99999999999995026, 8.999999999999992895 ) ) ;
#3071=ADVANCED_FACE ( 'NONE', ( #1325 ), #4185, .T. ) ;
#3075=EDGE_LOOP ( 'NONE', ( #1686, #3227, #1827, #2604 ) ) ;
#3077=LINE ( 'NONE', #110, #3278 ) ;
#3079=DIRECTION ( 'NONE',  ( 0.000000000000000000, -1.000000000000000000, 0.000000000000000000 ) ) ;
#3080=ORIENTED_EDGE ( 'NONE', *, *, #2078, .F. ) ;
#3085=CYLINDRICAL_SURFACE ( 'NONE', #4026, 3.999999999999998224 ) ;
#3094=ORIENTED_EDGE ( 'NONE', *, *, #230, .F. ) ;
#3095=ORIENTED_EDGE ( 'NONE', *, *, #1308, .F. ) ;
#3096=FACE_BOUND ( 'NONE', #4097, .T. ) ;
#3100=LINE ( 'NONE', #2346, #1834 ) ;
#3103=DIRECTION ( 'NONE',  ( -0.000000000000000000, -0.000000000000000000, 1.000000000000000000 ) ) ;
#3106=EDGE_CURVE ( 'NONE', #289, #181, #2869, .T. ) ;
#3107=CIRCLE ( 'NONE', #4321, 4.000000000000000000 ) ;
#3109=CARTESIAN_POINT ( 'NONE',  ( 20.46667490424620084, 21.93582988124910216, 12.87153294081770483 ) ) ;
#3110=( GEOMETRIC_REPRESENTATION_CONTEXT ( 3 ) GLOBAL_UNCERTAINTY_ASSIGNED_CONTEXT ( ( #1879 ) ) GLOBAL_UNIT_ASSIGNED_CONTEXT ( ( #2838, #2817, #657 ) ) REPRESENTATION_CONTEXT ( 'NONE', 'WORKASPACE' ) );
#3111=CARTESIAN_POINT ( 'NONE',  ( -27.10000000000000497, 0.6000000000000000888, 19.00000000000000000 ) ) ;
#3114=CARTESIAN_POINT ( 'NONE',  ( -20.50609665440989815, 14.84924240491747227, 8.999999999999992895 ) ) ;
#3116=VERTEX_POINT ( 'NONE', #3054 ) ;
#3117=AXIS2_PLACEMENT_3D ( 'NONE', #266, #290, #1783 ) ;
#3124=LINE ( 'NONE', #3522, #4050 ) ;
#3127=ADVANCED_FACE ( 'NONE', ( #4509 ), #1253, .T. ) ;
#3129=CARTESIAN_POINT ( 'NONE',  ( -3.999903055931597784, 29.73215053696358368, 8.737301635141733414 ) ) ;
#3131=DIRECTION ( 'NONE',  ( 1.000000000000000000, 0.000000000000000000, 0.000000000000000000 ) ) ;
#3132=EDGE_CURVE ( 'NONE', #4134, #2995, #245, .T. ) ;
#3136=DIRECTION ( 'NONE',  ( 1.000000000000000000, 0.000000000000000000, 0.000000000000000000 ) ) ;
#3138=VECTOR ( 'NONE', #3213, 1000.000000000000000 ) ;
#3150=ORIENTED_EDGE ( 'NONE', *, *, #3132, .T. ) ;
#3154=DIRECTION ( 'NONE',  ( -0.000000000000000000, -0.000000000000000000, 1.000000000000000000 ) ) ;
#3155=DIRECTION ( 'NONE',  ( 0.000000000000000000, 0.000000000000000000, 1.000000000000000000 ) ) ;
#3168=AXIS2_PLACEMENT_3D ( 'NONE', #4023, #3657, #4332 ) ;
#3169=CARTESIAN_POINT ( 'NONE',  ( 25.83240171513483929, 3.403349963601484340, 20.00001200000000168 ) ) ;
#3175=DIRECTION ( 'NONE',  ( -0.000000000000000000, -1.000000000000000000, -0.000000000000000000 ) ) ;
#3178=AXIS2_PLACEMENT_3D ( 'NONE', #3469, #2043, #547 ) ;
#3183=ORIENTED_EDGE ( 'NONE', *, *, #3267, .T. ) ;
#3185=CARTESIAN_POINT ( 'NONE',  ( -25.99307600111999150, 0.6000000000000000888, 20.00001200000000168 ) ) ;
#3189=ORIENTED_EDGE ( 'NONE', *, *, #2811, .T. ) ;
#3190=CARTESIAN_POINT ( 'NONE',  ( -0.5000000000000001110, 10.00000000000000000, 15.00000000000000178 ) ) ;
#3191=APPLICATION_CONTEXT ( 'automotive_design' ) ;
#3198=CARTESIAN_POINT ( 'NONE',  ( 26.00000000000000355, 1.592040838891558898E-15, 20.00000599999999906 ) ) ;
#3199=CARTESIAN_POINT ( 'NONE',  ( -23.83622240491805755, 18.21639843360778244, 8.473444514228551938 ) ) ;
#3200=CARTESIAN_POINT ( 'NONE',  ( 27.99999999999999645, 3.551475717527324030E-15, 20.00000000000000000 ) ) ;
#3206=DIRECTION ( 'NONE',  ( -1.000000000000000000, 0.000000000000000000, -0.000000000000000000 ) ) ;
#3213=DIRECTION ( 'NONE',  ( 0.000000000000000000, -1.000000000000000000, 0.000000000000000000 ) ) ;
#3214=DIRECTION ( 'NONE',  ( -0.7071067811865487940, 0.7071067811865463515, 0.000000000000000000 ) ) ;
#3215=EDGE_CURVE ( 'NONE', #2731, #741, #703, .T. ) ;
#3218=CARTESIAN_POINT ( 'NONE',  ( 2.004043995866382932, 29.93378982679665512, 12.47171604645195941 ) ) ;
#3222=AXIS2_PLACEMENT_3D ( 'NONE', #462, #3667, #4110 ) ;
#3224=DIRECTION ( 'NONE',  ( 0.000000000000000000, 0.000000000000000000, 1.000000000000000000 ) ) ;
#3227=ORIENTED_EDGE ( 'NONE', *, *, #2078, .T. ) ;
#3228=ORIENTED_EDGE ( 'NONE', *, *, #1404, .F. ) ;
#3231=SURFACE_STYLE_USAGE ( .BOTH. , #265 ) ;
#3237=DIRECTION ( 'NONE',  ( 0.000000000000000000, 0.000000000000000000, 1.000000000000000000 ) ) ;
#3250=DIRECTION ( 'NONE',  ( -0.000000000000000000, -0.000000000000000000, 1.000000000000000000 ) ) ;
#3253=VERTEX_POINT ( 'NONE', #1409 ) ;
#3259=ORIENTED_EDGE ( 'NONE', *, *, #778, .T. ) ;
#3267=EDGE_CURVE ( 'NONE', #2680, #2090, #2039, .T. ) ;
#3269=CARTESIAN_POINT ( 'NONE',  ( 22.10738654751468957, 20.28106296843835565, 5.205249767788495241 ) ) ;
#3270=DIRECTION ( 'NONE',  ( 1.000000000000000000, 0.000000000000000000, 0.000000000000000000 ) ) ;
#3277=VECTOR ( 'NONE', #4648, 1000.000000000000000 ) ;
#3278=VECTOR ( 'NONE', #534, 1000.000000000000000 ) ;
#3284=LINE ( 'NONE', #2880, #360 ) ;
#3285=CARTESIAN_POINT ( 'NONE',  ( -23.34243530581964166, 18.84548434425186869, 11.44084376890924304 ) ) ;
#3291=CARTESIAN_POINT ( 'NONE',  ( 20.46703030200860240, 21.93550942649225632, 5.128274502689554204 ) ) ;
#3292=AXIS2_PLACEMENT_3D ( 'NONE', #4364, #640, #3913 ) ;
#3293=CARTESIAN_POINT ( 'NONE',  ( 3.469446951953614189E-15, 30.00000000000000355, 4.999999999999992006 ) ) ;
#3307=CARTESIAN_POINT ( 'NONE',  ( -20.84186778456427902, 21.57966755480311960, 12.97440020260208193 ) ) ;
#3308=DIRECTION ( 'NONE',  ( 1.000000000000000000, 0.000000000000000000, 0.000000000000000000 ) ) ;
#3309=CARTESIAN_POINT ( 'NONE',  ( -23.36965697125209473, -11.52193136556785547, 20.00001200000000523 ) ) ;
#3314=DIRECTION ( 'NONE',  ( 0.7071067811865487940, -0.7071067811865463515, 0.000000000000000000 ) ) ;
#3318=ORIENTED_EDGE ( 'NONE', *, *, #363, .F. ) ;
#3325=ORIENTED_EDGE ( 'NONE', *, *, #3578, .F. ) ;
#3326=ORIENTED_EDGE ( 'NONE', *, *, #4639, .T. ) ;
#3328=DIRECTION ( 'NONE',  ( -0.7071067811865487940, -0.7071067811865463515, 0.000000000000000000 ) ) ;
#3329=CARTESIAN_POINT ( 'NONE',  ( -22.43321928693951506, 19.92007681871555036, 12.59316242105108508 ) ) ;
#3333=CARTESIAN_POINT ( 'NONE',  ( 11.52193136556785369, -23.36965697125208052, 20.00001199999999457 ) ) ;
#3339=AXIS2_PLACEMENT_3D ( 'NONE', #4540, #1657, #3513 ) ;
#3340=CARTESIAN_POINT ( 'NONE',  ( 19.74756467586676223, 22.58496929628982031, 5.529782636833618703 ) ) ;
#3341=CARTESIAN_POINT ( 'NONE',  ( 0.000000000000000000, 10.00000000000000000, 17.00000000000000000 ) ) ;
#3345=EDGE_LOOP ( 'NONE', ( #238, #2872, #4573, #1844 ) ) ;
#3349=CARTESIAN_POINT ( 'NONE',  ( -25.99307600111999150, 0.5999999999999998668, 19.00000000000000000 ) ) ;
#3351=ORIENTED_EDGE ( 'NONE', *, *, #2837, .T. ) ;
#3352=ORIENTED_EDGE ( 'NONE', *, *, #2646, .T. ) ;
#3359=CARTESIAN_POINT ( 'NONE',  ( -26.00000000000000355, -1.592040838891558504E-15, 20.00000599999999906 ) ) ;
#3361=VERTEX_POINT ( 'NONE', #1210 ) ;
#3362=CARTESIAN_POINT ( 'NONE',  ( 30.00000000000000355, 3.673940397442059967E-15, 20.00000000000000000 ) ) ;
#3367=DIRECTION ( 'NONE',  ( 0.000000000000000000, 0.000000000000000000, -1.000000000000000000 ) ) ;
#3375=ORIENTED_EDGE ( 'NONE', *, *, #1260, .T. ) ;
#3383=ORIENTED_EDGE ( 'NONE', *, *, #3939, .F. ) ;
#3386=DIRECTION ( 'NONE',  ( 0.000000000000000000, -1.000000000000000000, 0.000000000000000000 ) ) ;
#3387=CARTESIAN_POINT ( 'NONE',  ( -30.00000000000004974, 29.99999999999995737, 8.999999999999992895 ) ) ;
#3389=AXIS2_PLACEMENT_3D ( 'NONE', #1605, #1259, #1331 ) ;
#3393=EDGE_CURVE ( 'NONE', #2111, #2552, #3726, .T. ) ;
#3397=ORIENTED_EDGE ( 'NONE', *, *, #3741, .F. ) ;
#3400=PLANE ( 'NONE',  #4571 ) ;
#3403=EDGE_LOOP ( 'NONE', ( #2233, #1535, #1977, #2779 ) ) ;
#3404=ORIENTED_EDGE ( 'NONE', *, *, #987, .T. ) ;
#3405=DIRECTION ( 'NONE',  ( -0.7071067811865487940, -0.7071067811865463515, 0.000000000000000000 ) ) ;
#3406=CARTESIAN_POINT ( 'NONE',  ( 3.959305671612554781E-15, 25.00000000000000000, 12.99999999999999289 ) ) ;
#3408=CARTESIAN_POINT ( 'NONE',  ( -27.10000000000000497, -0.5999999999999998668, 19.59999999999999787 ) ) ;
#3413=ORIENTED_EDGE ( 'NONE', *, *, #2510, .F. ) ;
#3416=CARTESIAN_POINT ( 'NONE',  ( 19.41770456673556922, 22.86919556969938583, 12.17989986600643704 ) ) ;
#3419=CARTESIAN_POINT ( 'NONE',  ( -18.84457784187181062, 23.34316218245334795, 6.560806493199571321 ) ) ;
#3430=ORIENTED_EDGE ( 'NONE', *, *, #309, .F. ) ;
#3431=DIRECTION ( 'NONE',  ( 0.000000000000000000, 1.000000000000000000, 0.000000000000000000 ) ) ;
#3433=LINE ( 'NONE', #180, #2769 ) ;
#3436=AXIS2_PLACEMENT_3D ( 'NONE', #3053, #3431, #4083 ) ;
#3437=ADVANCED_FACE ( 'NONE', ( #2334 ), #3085, .F. ) ;
#3438=CARTESIAN_POINT ( 'NONE',  ( 3.959305739469038251E-15, 30.00000000000000355, 12.99999999999999289 ) ) ;
#3444=ORIENTED_EDGE ( 'NONE', *, *, #2837, .F. ) ;
#3463=CARTESIAN_POINT ( 'NONE',  ( -4.000096396247766251, 29.73212452601126188, 9.259737768674039415 ) ) ;
#3469=CARTESIAN_POINT ( 'NONE',  ( 0.000000000000000000, 0.000000000000000000, 19.00000000000000000 ) ) ;
#3471=EDGE_LOOP ( 'NONE', ( #500, #1589, #513, #1255 ) ) ;
#3472=VERTEX_POINT ( 'NONE', #977 ) ;
#3474=FACE_OUTER_BOUND ( 'NONE', #239, .T. ) ;
#3476=DIRECTION ( 'NONE',  ( 1.000000000000000000, 0.000000000000000000, 0.000000000000000000 ) ) ;
#3477=VERTEX_POINT ( 'NONE', #3512 ) ;
#3487=MECHANICAL_DESIGN_GEOMETRIC_PRESENTATION_REPRESENTATION('',(#606),#3110);
#3489=CARTESIAN_POINT ( 'NONE',  ( -22.10500230410275790, 20.28368189782978703, 5.203924605526645486 ) ) ;
#3491=CARTESIAN_POINT ( 'NONE',  ( 0.000000000000000000, 0.000000000000000000, 0.000000000000000000 ) ) ;
#3494=VERTEX_POINT ( 'NONE', #3114 ) ;
#3502=LINE ( 'NONE', #4582, #1855 ) ;
#3506=AXIS2_PLACEMENT_3D ( 'NONE', #2158, #2116, #4 ) ;
#3511=CARTESIAN_POINT ( 'NONE',  ( -23.60249532755124591, 18.51843501006184312, 7.226626843687534496 ) ) ;
#3512=CARTESIAN_POINT ( 'NONE',  ( -24.00000000000000355, 2.939152317953648289E-15, 19.00000000000000000 ) ) ;
#3513=DIRECTION ( 'NONE',  ( 1.000000000000000000, 0.000000000000000000, 0.000000000000000000 ) ) ;
#3514=VERTEX_POINT ( 'NONE', #3874 ) ;
#3518=( LENGTH_UNIT ( ) NAMED_UNIT ( * ) SI_UNIT ( .MILLI., .METRE. ) );
#3520=CARTESIAN_POINT ( 'NONE',  ( 1.701696020694463574, 25.99999999999999645, 20.00001200000000168 ) ) ;
#3522=CARTESIAN_POINT ( 'NONE',  ( -32.82842712474623426, 27.17157287525376219, 8.999999999999992895 ) ) ;
#3525=CARTESIAN_POINT ( 'NONE',  ( 4.000183053129181765, 29.73211286767113037, 8.738350868772759128 ) ) ;
#3527=CIRCLE ( 'NONE', #1779, 0.5000000000000001110 ) ;
#3528=CIRCLE ( 'NONE', #122, 30.00000000000000355 ) ;
#3529=CARTESIAN_POINT ( 'NONE',  ( 23.85222316637486273, 18.19536891688240843, 8.999999999999992895 ) ) ;
#3530=CARTESIAN_POINT ( 'NONE',  ( -23.85222316637485562, 18.19536891688241198, 8.999999999999992895 ) ) ;
#3537=B_SPLINE_CURVE_WITH_KNOTS ( 'NONE', 3,
 ( #2836, #271, #4705, #315, #295, #4248, #3218, #2147, #1742, #3964, #1389, #2100, #991, #4657, #3885, #4296, #2421, #3525, #2860, #704, #634, #3547, #1033, #2518, #2442, #2791, #339, #2882, #4681, #4631, #1009, #2125, #2814, #1348 ),
 .UNSPECIFIED., .F., .F.,
 ( 4, 2, 2, 2, 2, 2, 2, 2, 2, 2, 2, 2, 2, 2, 2, 2, 4 ),
 ( 0.01251976117704806969, 0.01330205745918825073, 0.01408435374132843351, 0.01486665002346861456, 0.01564894630560879560, 0.01643124258774897664, 0.01721353886988916115, 0.01799583515202934220, 0.01877813143416952324, 0.01956042771630970428, 0.02034272399844988533, 0.02112502028059006637, 0.02190731656273024741, 0.02268961284487042845, 0.02347190912701060950, 0.02425420540915079401, 0.02503650169129097505 ),
 .UNSPECIFIED. ) ;
#3540=CARTESIAN_POINT ( 'NONE',  ( 17.67766952966372429, 17.67766952966365679, 8.999999999999992895 ) ) ;
#3543=EDGE_LOOP ( 'NONE', ( #2198, #2949, #272, #1729 ) ) ;
#3544=CARTESIAN_POINT ( 'NONE',  ( -27.10000000000000497, -0.5999999999999998668, 19.59999999999999787 ) ) ;
#3547=CARTESIAN_POINT ( 'NONE',  ( 3.595673326866945629, 29.78391060080977226, 7.228055294346797943 ) ) ;
#3549=VECTOR ( 'NONE', #679, 1000.000000000000000 ) ;
#3551=CARTESIAN_POINT ( 'NONE',  ( 8.377607117416804527, -24.67207871933483787, 20.00001200000000168 ) ) ;
#3553=EDGE_CURVE ( 'NONE', #3494, #2903, #3669, .T. ) ;
#3554=DIRECTION ( 'NONE',  ( 0.7071067811865487940, 0.7071067811865463515, 0.000000000000000000 ) ) ;
#3556=CYLINDRICAL_SURFACE ( 'NONE', #421, 8.000000000000000000 ) ;
#3558=EDGE_LOOP ( 'NONE', ( #452, #2709, #3832, #1405 ) ) ;
#3569=CARTESIAN_POINT ( 'NONE',  ( -0.7500000000000001110, 9.184850993605150903E-17, 17.00000000000000000 ) ) ;
#3571=CARTESIAN_POINT ( 'NONE',  ( 0.000000000000000000, 0.000000000000000000, 15.00000000000000178 ) ) ;
#3578=EDGE_CURVE ( 'NONE', #4099, #4118, #950, .T. ) ;
#3582=VECTOR ( 'NONE', #4234, 1000.000000000000000 ) ;
#3584=ORIENTED_EDGE ( 'NONE', *, *, #1034, .F. ) ;
#3585=EDGE_LOOP ( 'NONE', ( #2250, #1852, #3728, #2266 ) ) ;
#3589=SURFACE_STYLE_FILL_AREA ( #984 ) ;
#3592=FACE_OUTER_BOUND ( 'NONE', #2526, .T. ) ;
#3594=CARTESIAN_POINT ( 'NONE',  ( -27.17157287525386877, 32.82842712474614899, 8.999999999999992895 ) ) ;
#3597=DIRECTION ( 'NONE',  ( 0.000000000000000000, -0.000000000000000000, -1.000000000000000000 ) ) ;
#3602=AXIS2_PLACEMENT_3D ( 'NONE', #1395, #3224, #3270 ) ;
#3606=DIRECTION ( 'NONE',  ( -0.000000000000000000, -0.000000000000000000, 1.000000000000000000 ) ) ;
#3609=ORIENTED_EDGE ( 'NONE', *, *, #2811, .F. ) ;
#3616=VECTOR ( 'NONE', #3059, 1000.000000000000000 ) ;
#3624=CARTESIAN_POINT ( 'NONE',  ( 23.83634335050103203, 18.21624151457274365, 9.526033398219871273 ) ) ;
#3626=CARTESIAN_POINT ( 'NONE',  ( 0.000000000000000000, 0.000000000000000000, 20.00000000000000000 ) ) ;
#3628=AXIS2_PLACEMENT_3D ( 'NONE', #884, #1572, #3023 ) ;
#3629=LINE ( 'NONE', #1439, #4373 ) ;
#3642=FACE_BOUND ( 'NONE', #549, .T. ) ;
#3648=PRODUCT_DEFINITION ( 'UNKNOWN', '', #4612, #2809 ) ;
#3649=CARTESIAN_POINT ( 'NONE',  ( 23.85222316637486273, 18.19536891688240843, 8.999999999999992895 ) ) ;
#3652=ORIENTED_EDGE ( 'NONE', *, *, #4064, .F. ) ;
#3657=DIRECTION ( 'NONE',  ( 0.000000000000000000, 0.000000000000000000, -1.000000000000000000 ) ) ;
#3662=DIRECTION ( 'NONE',  ( -0.7071067811865487940, -0.7071067811865463515, 0.000000000000000000 ) ) ;
#3663=CARTESIAN_POINT ( 'NONE',  ( -18.36067068532948099, 23.72542776831230071, 10.29518969959635299 ) ) ;
#3664=CARTESIAN_POINT ( 'NONE',  ( 3.469446951953614189E-15, 25.00000000000000000, 4.999999999999992006 ) ) ;
#3665=CARTESIAN_POINT ( 'NONE',  ( 25.16843286583315020, -6.741346781237215424, 20.00001200000000168 ) ) ;
#3667=DIRECTION ( 'NONE',  ( 1.000000000000000000, -0.000000000000000000, 0.000000000000000000 ) ) ;
#3668=CARTESIAN_POINT ( 'NONE',  ( 23.34316218245341190, 18.84457784187173246, 6.560806493199571321 ) ) ;
#3669=CIRCLE ( 'NONE', #409, 4.000000000000000000 ) ;
#3670=CARTESIAN_POINT ( 'NONE',  ( -3.595210675795415867, 29.78396494222454294, 7.227341970420264161 ) ) ;
#3682=VERTEX_POINT ( 'NONE', #4707 ) ;
#3684=CARTESIAN_POINT ( 'NONE',  ( -23.85222316637485562, 18.19536891688241198, 8.999999999999992895 ) ) ;
#3686=CARTESIAN_POINT ( 'NONE',  ( -26.00000000000000355, -1.701696020694477784, 20.00001200000000523 ) ) ;
#3699=EDGE_LOOP ( 'NONE', ( #802, #2557 ) ) ;
#3700=EDGE_CURVE ( 'NONE', #2552, #2995, #1064, .T. ) ;
#3706=VERTEX_POINT ( 'NONE', #3200 ) ;
#3718=AXIS2_PLACEMENT_3D ( 'NONE', #1618, #649, #3206 ) ;
#3726=LINE ( 'NONE', #471, #1283 ) ;
#3728=ORIENTED_EDGE ( 'NONE', *, *, #390, .F. ) ;
#3734=CARTESIAN_POINT ( 'NONE',  ( -20.28376480839715157, 22.10492369241840649, 12.79609622574099070 ) ) ;
#3741=EDGE_CURVE ( 'NONE', #1957, #3924, #4679, .T. ) ;
#3745=CARTESIAN_POINT ( 'NONE',  ( -1.290629128713961293, 29.97320584640673147, 5.204870533884474071 ) ) ;
#3746=DIRECTION ( 'NONE',  ( -1.000000000000000000, 0.000000000000000000, 0.000000000000000000 ) ) ;
#3757=CARTESIAN_POINT ( 'NONE',  ( -24.00000000000000355, 2.939152317953648289E-15, 17.00000000000000000 ) ) ;
#3763=DIRECTION ( 'NONE',  ( 0.000000000000000000, 0.000000000000000000, -1.000000000000000000 ) ) ;
#3768=DIRECTION ( 'NONE',  ( 0.000000000000000000, 0.000000000000000000, -1.000000000000000000 ) ) ;
#3774=PRODUCT ( 'casing', 'casing', '', ( #4035 ) ) ;
#3780=CARTESIAN_POINT ( 'NONE',  ( -21.02743970908340287, 21.39894891851812986, 5.000096751259999195 ) ) ;
#3783=ORIENTED_EDGE ( 'NONE', *, *, #1517, .T. ) ;
#3795=DIRECTION ( 'NONE',  ( -1.000000000000000000, -0.000000000000000000, -0.000000000000000000 ) ) ;
#3808=DIRECTION ( 'NONE',  ( -1.000000000000000000, 0.000000000000000000, 0.000000000000000000 ) ) ;
#3811=EDGE_LOOP ( 'NONE', ( #4400, #2457, #3150, #623 ) ) ;
#3815=DIRECTION ( 'NONE',  ( 1.000000000000000000, 0.000000000000000000, 0.000000000000000000 ) ) ;
#3823=CARTESIAN_POINT ( 'NONE',  ( -2.440392720584789288, 29.90136469312441037, 12.17998752022640296 ) ) ;
#3824=CARTESIAN_POINT ( 'NONE',  ( 3.469446951953614189E-15, 25.00000000000000000, 8.999999999999992895 ) ) ;
#3826=DIRECTION ( 'NONE',  ( -0.7071067811865487940, 0.7071067811865463515, 0.000000000000000000 ) ) ;
#3827=CARTESIAN_POINT ( 'NONE',  ( -25.16843286583315731, 6.741346781237202102, 20.00001200000000168 ) ) ;
#3831=ADVANCED_FACE ( 'NONE', ( #4039 ), #115, .F. ) ;
#3832=ORIENTED_EDGE ( 'NONE', *, *, #2510, .T. ) ;
#3833=LINE ( 'NONE', #3185, #2406 ) ;
#3834=EDGE_CURVE ( 'NONE', #1513, #956, #3988, .T. ) ;
#3838=CARTESIAN_POINT ( 'NONE',  ( 0.000000000000000000, 0.000000000000000000, 17.99999999999998579 ) ) ;
#3839=ORIENTED_EDGE ( 'NONE', *, *, #3956, .T. ) ;
#3840=CIRCLE ( 'NONE', #4365, 26.00000000000000355 ) ;
#3847=CARTESIAN_POINT ( 'NONE',  ( 21.02424009228912993, 21.40213195504970756, 12.99981531858142425 ) ) ;
#3850=AXIS2_PLACEMENT_3D ( 'NONE', #4136, #3155, #3131 ) ;
#3851=FACE_OUTER_BOUND ( 'NONE', #3585, .T. ) ;
#3854=CARTESIAN_POINT ( 'NONE',  ( 0.5000000000000001110, 10.00000000000000000, 15.00000000000000178 ) ) ;
#3857=EDGE_CURVE ( 'NONE', #2030, #2679, #708, .T. ) ;
#3860=FACE_OUTER_BOUND ( 'NONE', #204, .T. ) ;
#3865=DIRECTION ( 'NONE',  ( 1.000000000000000000, 0.000000000000000000, 0.000000000000000000 ) ) ;
#3870=CARTESIAN_POINT ( 'NONE',  ( 21.93211642885839296, 20.47065640071369685, 12.87299606428841159 ) ) ;
#3874=CARTESIAN_POINT ( 'NONE',  ( 0.7500000000000001110, 0.000000000000000000, 15.00000000000000178 ) ) ;
#3885=CARTESIAN_POINT ( 'NONE',  ( 3.871533456320507494, 29.74918284297944382, 10.03884696677421395 ) ) ;
#3890=AXIS2_PLACEMENT_3D ( 'NONE', #1872, #2246, #4092 ) ;
#3891=AXIS2_PLACEMENT_3D ( 'NONE', #1503, #779, #2240 ) ;
#3893=CYLINDRICAL_SURFACE ( 'NONE', #4004, 0.5000000000000001110 ) ;
#3896=CARTESIAN_POINT ( 'NONE',  ( -27.10000000000000497, -0.5999999999999998668, 19.59999999999999787 ) ) ;
#3898=ORIENTED_EDGE ( 'NONE', *, *, #390, .T. ) ;
#3907=PLANE ( 'NONE',  #797 ) ;
#3908=ORIENTED_EDGE ( 'NONE', *, *, #724, .T. ) ;
#3913=DIRECTION ( 'NONE',  ( -1.000000000000000000, 0.000000000000000000, 0.000000000000000000 ) ) ;
#3914=EDGE_CURVE ( 'NONE', #3514, #907, #1258, .T. ) ;
#3916=CARTESIAN_POINT ( 'NONE',  ( 20.67279826512042362, -15.85973458909328571, 20.00001200000000523 ) ) ;
#3917=EDGE_CURVE ( 'NONE', #3361, #1928, #871, .T. ) ;
#3922=CIRCLE ( 'NONE', #3009, 4.000000000000000000 ) ;
#3924=VERTEX_POINT ( 'NONE', #2864 ) ;
#3925=VERTEX_POINT ( 'NONE', #299 ) ;
#3928=DIRECTION ( 'NONE',  ( -1.000000000000000000, 0.000000000000000000, 0.000000000000000000 ) ) ;
#3933=EDGE_LOOP ( 'NONE', ( #550, #4395 ) ) ;
#3937=FACE_OUTER_BOUND ( 'NONE', #2245, .T. ) ;
#3938=ADVANCED_FACE ( 'NONE', ( #1414, #2547 ), #2447, .T. ) ;
#3939=EDGE_CURVE ( 'NONE', #4187, #3116, #647, .T. ) ;
#3945=CARTESIAN_POINT ( 'NONE',  ( -23.23798364781088210, 18.97448886297816273, 6.357861838490105555 ) ) ;
#3956=EDGE_CURVE ( 'NONE', #4460, #2036, #650, .T. ) ;
#3957=DIRECTION ( 'NONE',  ( 1.000000000000000000, 0.000000000000000000, 0.000000000000000000 ) ) ;
#3960=CARTESIAN_POINT ( 'NONE',  ( 26.00000000000000355, 1.592040838891558898E-15, 20.00000599999999906 ) ) ;
#3962=DIRECTION ( 'NONE',  ( 0.000000000000000000, 0.000000000000000000, 1.000000000000000000 ) ) ;
#3964=CARTESIAN_POINT ( 'NONE',  ( 3.011018170818868800, 29.84908880846061408, 11.64607938208749971 ) ) ;
#3967=CARTESIAN_POINT ( 'NONE',  ( 0.000000000000000000, 0.000000000000000000, 19.59999999999999787 ) ) ;
#3969=DIRECTION ( 'NONE',  ( -0.7071067811865456854, 0.000000000000000000, -0.7071067811865493491 ) ) ;
#3974=ORIENTED_EDGE ( 'NONE', *, *, #2773, .T. ) ;
#3975=CYLINDRICAL_SURFACE ( 'NONE', #843, 26.00000000000000355 ) ;
#3980=CARTESIAN_POINT ( 'NONE',  ( 11.52193136556786257, 23.36965697125208052, 20.00001200000000168 ) ) ;
#3986=CARTESIAN_POINT ( 'NONE',  ( 22.86660962422647358, 19.42075468095221424, 12.18297904795690378 ) ) ;
#3988=CIRCLE ( 'NONE', #4599, 8.000000000000000000 ) ;
#3998=AXIS2_PLACEMENT_3D ( 'NONE', #2942, #1506, #3746 ) ;
#4004=AXIS2_PLACEMENT_3D ( 'NONE', #4054, #406, #59 ) ;
#4014=CARTESIAN_POINT ( 'NONE',  ( 23.72646225117223295, 18.35933649373362897, 7.709376215153276313 ) ) ;
#4021=DIRECTION ( 'NONE',  ( -0.7071067811865487940, 0.7071067811865463515, 0.000000000000000000 ) ) ;
#4023=CARTESIAN_POINT ( 'NONE',  ( 0.000000000000000000, 0.000000000000000000, 19.59999999999999787 ) ) ;
#4024=EDGE_LOOP ( 'NONE', ( #3430, #4377 ) ) ;
#4026=AXIS2_PLACEMENT_3D ( 'NONE', #1333, #903, #2701 ) ;
#4029=CARTESIAN_POINT ( 'NONE',  ( -19.92389804225928529, 22.42982507849018958, 12.59566700906149173 ) ) ;
#4030=CARTESIAN_POINT ( 'NONE',  ( 0.000000000000000000, 0.000000000000000000, 20.00000000000000000 ) ) ;
#4031=CARTESIAN_POINT ( 'NONE',  ( 6.741346781237209207, -25.16843286583315731, 20.00001199999999812 ) ) ;
#4032=EDGE_LOOP ( 'NONE', ( #44, #354, #217, #350 ) ) ;
#4033=CARTESIAN_POINT ( 'NONE',  ( -30.00000000000000355, 0.000000000000000000, 0.000000000000000000 ) ) ;
#4034=FACE_OUTER_BOUND ( 'NONE', #1219, .T. ) ;
#4035=PRODUCT_CONTEXT ( 'NONE', #4178, 'mechanical' ) ;
#4039=FACE_OUTER_BOUND ( 'NONE', #169, .T. ) ;
#4045=AXIS2_PLACEMENT_3D ( 'NONE', #278, #3554, #1394 ) ;
#4047=EDGE_LOOP ( 'NONE', ( #4349, #3444, #4542, #2067 ) ) ;
#4049=ORIENTED_EDGE ( 'NONE', *, *, #230, .T. ) ;
#4050=VECTOR ( 'NONE', #944, 1000.000000000000000 ) ;
#4054=CARTESIAN_POINT ( 'NONE',  ( 0.000000000000000000, 10.00000000000000000, 13.00000000000000178 ) ) ;
#4061=CARTESIAN_POINT ( 'NONE',  ( 22.87032942663243773, 19.41638709359441606, 5.821272343678753458 ) ) ;
#4064=EDGE_CURVE ( 'NONE', #305, #4187, #3840, .T. ) ;
#4071=FACE_OUTER_BOUND ( 'NONE', #1569, .T. ) ;
#4072=ORIENTED_EDGE ( 'NONE', *, *, #189, .F. ) ;
#4077=CARTESIAN_POINT ( 'NONE',  ( -18.21624151457282537, 23.83634335050096809, 9.526033398219878379 ) ) ;
#4078=LINE ( 'NONE', #108, #2308 ) ;
#4079=DIRECTION ( 'NONE',  ( 1.000000000000000000, 0.000000000000000000, -0.000000000000000000 ) ) ;
#4083=DIRECTION ( 'NONE',  ( 0.000000000000000000, 0.000000000000000000, 1.000000000000000000 ) ) ;
#4087=CARTESIAN_POINT ( 'NONE',  ( 18.19536891688250435, 23.85222316637480944, 8.738792385868094925 ) ) ;
#4092=DIRECTION ( 'NONE',  ( -1.000000000000000000, 0.000000000000000000, -0.000000000000000000 ) ) ;
#4093=AXIS2_PLACEMENT_3D ( 'NONE', #338, #2813, #3865 ) ;
#4095=ADVANCED_FACE ( 'NONE', ( #4414 ), #436, .F. ) ;
#4097=EDGE_LOOP ( 'NONE', ( #1314, #561 ) ) ;
#4099=VERTEX_POINT ( 'NONE', #775 ) ;
#4105=EDGE_CURVE ( 'NONE', #2482, #2135, #3527, .T. ) ;
#4107=CYLINDRICAL_SURFACE ( 'NONE', #2164, 30.00000000000000355 ) ;
#4110=DIRECTION ( 'NONE',  ( 0.000000000000000000, 0.000000000000000000, -1.000000000000000000 ) ) ;
#4112=CARTESIAN_POINT ( 'NONE',  ( 0.000000000000000000, 0.000000000000000000, 17.00000000000000000 ) ) ;
#4115=CARTESIAN_POINT ( 'NONE',  ( 0.000000000000000000, 0.000000000000000000, 20.00000000000000000 ) ) ;
#4118=VERTEX_POINT ( 'NONE', #2937 ) ;
#4123=AXIS2_PLACEMENT_3D ( 'NONE', #1562, #4470, #1209 ) ;
#4125=CARTESIAN_POINT ( 'NONE',  ( -21.02820489033399554, 21.39823644064415120, 13.00018275065233020 ) ) ;
#4133=FACE_BOUND ( 'NONE', #3699, .T. ) ;
#4134=VERTEX_POINT ( 'NONE', #1528 ) ;
#4136=CARTESIAN_POINT ( 'NONE',  ( 0.000000000000000000, 0.000000000000000000, 15.00000000000000178 ) ) ;
#4139=CARTESIAN_POINT ( 'NONE',  ( -19.74853269256677990, 22.58414294016069945, 5.528858171306252345 ) ) ;
#4148=LINE ( 'NONE', #602, #539 ) ;
#4155=DIRECTION ( 'NONE',  ( -0.000000000000000000, -0.000000000000000000, 1.000000000000000000 ) ) ;
#4156=DIRECTION ( 'NONE',  ( 0.000000000000000000, 0.000000000000000000, 1.000000000000000000 ) ) ;
#4160=EDGE_LOOP ( 'NONE', ( #1214, #3375, #4476, #811, #3094, #2009, #2593, #2611 ) ) ;
#4162=ADVANCED_FACE ( 'NONE', ( #4034 ), #2212, .T. ) ;
#4165=CARTESIAN_POINT ( 'NONE',  ( -3.871674220476135631, 29.74916513505594295, 7.961019890438434388 ) ) ;
#4167=CARTESIAN_POINT ( 'NONE',  ( -20.84134157445931734, 21.58020450303982329, 5.025533726064749906 ) ) ;
#4170=CARTESIAN_POINT ( 'NONE',  ( -15.85973458909327860, 20.67279826512041652, 20.00001200000000168 ) ) ;
#4173=ORIENTED_EDGE ( 'NONE', *, *, #3917, .F. ) ;
#4178=APPLICATION_CONTEXT ( 'automotive_design' ) ;
#4185=PLANE ( 'NONE',  #368 ) ;
#4186=CARTESIAN_POINT ( 'NONE',  ( 0.000000000000000000, 0.000000000000000000, 17.00000000000000000 ) ) ;
#4187=VERTEX_POINT ( 'NONE', #111 ) ;
#4194=DIRECTION ( 'NONE',  ( 0.000000000000000000, 0.000000000000000000, 1.000000000000000000 ) ) ;
#4196=ORIENTED_EDGE ( 'NONE', *, *, #722, .F. ) ;
#4200=ORIENTED_EDGE ( 'NONE', *, *, #778, .F. ) ;
#4204=CONICAL_SURFACE ( 'NONE', #1069, 27.99999999999999645, 0.7853981633974457255 ) ;
#4207=CYLINDRICAL_SURFACE ( 'NONE', #1257, 4.000000000000000000 ) ;
#4211=CARTESIAN_POINT ( 'NONE',  ( 18.35919055844633974, 23.72657184721635204, 10.28976100101469981 ) ) ;
#4212=EDGE_CURVE ( 'NONE', #2030, #4484, #4510, .T. ) ;
#4214=CARTESIAN_POINT ( 'NONE',  ( -20.28106296843844092, 22.10738654751461851, 5.205249767788494353 ) ) ;
#4222=DIRECTION ( 'NONE',  ( -0.000000000000000000, -0.000000000000000000, 1.000000000000000000 ) ) ;
#4227=CARTESIAN_POINT ( 'NONE',  ( 3.469446951953614189E-15, 30.00000000000000355, 4.999999999999992006 ) ) ;
#4228=ORIENTED_EDGE ( 'NONE', *, *, #1748, .T. ) ;
#4231=CARTESIAN_POINT ( 'NONE',  ( 21.57966755480319421, 20.84186778456420797, 12.97440020260208193 ) ) ;
#4232=CARTESIAN_POINT ( 'NONE',  ( 27.09999999999999787, -0.5999999999999998668, 19.59999999999999787 ) ) ;
#4234=DIRECTION ( 'NONE',  ( -0.000000000000000000, -1.000000000000000000, -0.000000000000000000 ) ) ;
#4240=PLANE ( 'NONE',  #1655 ) ;
#4243=ADVANCED_FACE ( 'NONE', ( #1649 ), #4207, .F. ) ;
#4244=DIRECTION ( 'NONE',  ( -0.000000000000000000, 1.000000000000000000, 0.000000000000000000 ) ) ;
#4247=AXIS2_PLACEMENT_3D ( 'NONE', #3069, #3328, #4524 ) ;
#4248=CARTESIAN_POINT ( 'NONE',  ( 1.771177265432712700, 29.94863972218313464, 12.59594310203364387 ) ) ;
#4252=CARTESIAN_POINT ( 'NONE',  ( -3.796077574538131660, 29.75903253174124430, 10.28786097927510923 ) ) ;
#4253=AXIS2_PLACEMENT_3D ( 'NONE', #179, #585, #4581 ) ;
#4254=CARTESIAN_POINT ( 'NONE',  ( 24.67207871933483432, -8.377607117416795646, 20.00001200000000523 ) ) ;
#4257=LINE ( 'NONE', #3896, #2699 ) ;
#4259=ORIENTED_EDGE ( 'NONE', *, *, #2377, .F. ) ;
#4268=DIRECTION ( 'NONE',  ( -1.000000000000000000, -0.000000000000000000, -0.000000000000000000 ) ) ;
#4270=FACE_OUTER_BOUND ( 'NONE', #383, .T. ) ;
#4279=VECTOR ( 'NONE', #789, 1000.000000000000000 ) ;
#4280=CARTESIAN_POINT ( 'NONE',  ( -22.99914926278833249, 19.26328748721751438, 5.984828968106582714 ) ) ;
#4284=ORIENTED_EDGE ( 'NONE', *, *, #309, .T. ) ;
#4286=CYLINDRICAL_SURFACE ( 'NONE', #1359, 24.00000000000000355 ) ;
#4287=EDGE_CURVE ( 'NONE', #3116, #3925, #3502, .T. ) ;
#4289=CARTESIAN_POINT ( 'NONE',  ( 0.000000000000000000, 0.000000000000000000, 0.000000000000000000 ) ) ;
#4296=CARTESIAN_POINT ( 'NONE',  ( 3.973627609689486917, 29.73571816432124493, 9.527501605019752517 ) ) ;
#4303=ADVANCED_FACE ( 'NONE', ( #4133, #536, #226 ), #2719, .T. ) ;
#4312=CIRCLE ( 'NONE', #2785, 0.5000000000000001110 ) ;
#4318=CARTESIAN_POINT ( 'NONE',  ( -27.10000000000000497, 0.6000000000000000888, 19.59999999999999787 ) ) ;
#4321=AXIS2_PLACEMENT_3D ( 'NONE', #3540, #2411, #1687 ) ;
#4323=CARTESIAN_POINT ( 'NONE',  ( -23.72677024356903530, 18.35893773391720529, 7.710863047761279176 ) ) ;
#4325=DIRECTION ( 'NONE',  ( 1.000000000000000000, 0.000000000000000000, 0.000000000000000000 ) ) ;
#4330=CARTESIAN_POINT ( 'NONE',  ( 14.84924240491753800, 20.50609665440984841, 8.999999999999992895 ) ) ;
#4331=( NAMED_UNIT ( * ) SI_UNIT ( $, .STERADIAN. ) SOLID_ANGLE_UNIT ( ) );
#4332=DIRECTION ( 'NONE',  ( -1.000000000000000000, 0.000000000000000000, 0.000000000000000000 ) ) ;
#4335=PLANE ( 'NONE',  #2184 ) ;
#4336=CIRCLE ( 'NONE', #4343, 4.000000000000000000 ) ;
#4338=DIRECTION ( 'NONE',  ( 1.000000000000000000, 0.000000000000000000, 0.000000000000000000 ) ) ;
#4339=EDGE_CURVE ( 'NONE', #4118, #1513, #3433, .T. ) ;
#4341=CARTESIAN_POINT ( 'NONE',  ( 22.58188871325897296, 19.75109744359741981, 12.47298490618377720 ) ) ;
#4343=AXIS2_PLACEMENT_3D ( 'NONE', #470, #4021, #2199 ) ;
#4347=CLOSED_SHELL ( 'NONE', ( #1280, #4473, #4243, #4095, #3437, #2289, #1878, #392, #2750, #1417, #332, #3831, #4303, #4487, #3044, #4430, #3127, #891, #4655, #2722, #2388, #2502, #1155, #2688, #254, #1215, #914, #624, #1583, #3938, #4162, #1495, #193, #3071, #1617, #1378, #112, #4411 ) ) ;
#4349=ORIENTED_EDGE ( 'NONE', *, *, #2027, .F. ) ;
#4360=FACE_BOUND ( 'NONE', #1576, .T. ) ;
#4364=CARTESIAN_POINT ( 'NONE',  ( 0.000000000000000000, 0.000000000000000000, 19.59999999999999787 ) ) ;
#4365=AXIS2_PLACEMENT_3D ( 'NONE', #4463, #1888, #2961 ) ;
#4373=VECTOR ( 'NONE', #3606, 1000.000000000000000 ) ;
#4377=ORIENTED_EDGE ( 'NONE', *, *, #974, .F. ) ;
#4381=CARTESIAN_POINT ( 'NONE',  ( -22.10831845702707454, 20.28006516365564238, 12.79440425686131988 ) ) ;
#4384=EDGE_CURVE ( 'NONE', #2679, #2030, #3537, .T. ) ;
#4386=CARTESIAN_POINT ( 'NONE',  ( -25.83240171513484285, -3.403349963601435935, 20.00001200000000168 ) ) ;
#4390=CARTESIAN_POINT ( 'NONE',  ( 21.02954719696287356, 21.39687781493357832, 4.999903794384585431 ) ) ;
#4394=ORIENTED_EDGE ( 'NONE', *, *, #1910, .F. ) ;
#4395=ORIENTED_EDGE ( 'NONE', *, *, #4384, .F. ) ;
#4399=CARTESIAN_POINT ( 'NONE',  ( 3.469446951953614189E-15, 30.00000000000000355, 8.999999999999992895 ) ) ;
#4400=ORIENTED_EDGE ( 'NONE', *, *, #3393, .F. ) ;
#4404=LINE ( 'NONE', #3594, #1285 ) ;
#4408=CARTESIAN_POINT ( 'NONE',  ( -11.52193136556784658, -23.36965697125209118, 20.00001200000000168 ) ) ;
#4411=ADVANCED_FACE ( 'NONE', ( #4270 ), #3907, .T. ) ;
#4414=FACE_OUTER_BOUND ( 'NONE', #1514, .T. ) ;
#4416=CARTESIAN_POINT ( 'NONE',  ( 20.28368189782986519, 22.10500230410270106, 5.203924605526645486 ) ) ;
#4429=CARTESIAN_POINT ( 'NONE',  ( -21.93582988124917321, 20.46667490424612268, 12.87153294081770483 ) ) ;
#4430=ADVANCED_FACE ( 'NONE', ( #3937 ), #681, .F. ) ;
#4431=CARTESIAN_POINT ( 'NONE',  ( -0.7500000000000001110, 9.184850993605150903E-17, 15.00000000000000178 ) ) ;
#4438=CARTESIAN_POINT ( 'NONE',  ( 18.35893773391728701, 23.72677024356898201, 7.710863047761277400 ) ) ;
#4443=ORIENTED_EDGE ( 'NONE', *, *, #3393, .T. ) ;
#4445=AXIS2_PLACEMENT_3D ( 'NONE', #3967, #2886, #1014 ) ;
#4456=CARTESIAN_POINT ( 'NONE',  ( 27.17157287525387588, 32.82842712474614189, 8.999999999999992895 ) ) ;
#4460=VERTEX_POINT ( 'NONE', #1496 ) ;
#4461=VECTOR ( 'NONE', #594, 1000.000000000000000 ) ;
#4463=CARTESIAN_POINT ( 'NONE',  ( 0.000000000000000000, 0.000000000000000000, 19.59999999999999787 ) ) ;
#4464=B_SPLINE_CURVE_WITH_KNOTS ( 'NONE', 3,
 ( #1584, #1309, #1992, #519, #4492, #185, #567, #3419, #2751, #1262, #2312, #4139, #2700, #4214, #875, #4167, #3780, #2380, #595, #2040, #3489, #2106, #301, #1418, #4280, #3945, #1771, #665, #3511, #4323, #1751, #3199, #1017, #618 ),
 .UNSPECIFIED., .F., .F.,
 ( 4, 2, 2, 2, 2, 2, 2, 2, 2, 2, 2, 2, 2, 2, 2, 2, 4 ),
 ( 0.000000000000000000, 0.0007824845743203488312, 0.001564969148640697662, 0.002347453722961046277, 0.003129938297281395325, 0.003912422871601744373, 0.004694907445922092554, 0.005477392020242441602, 0.006259876594562790650, 0.007042361168883139698, 0.007824845743203488746, 0.008607330317523836927, 0.009389814891844185107, 0.01017229946616453502, 0.01095478404048488320, 0.01173726861480523312, 0.01251975318912558130 ),
 .UNSPECIFIED. ) ;
#4468=VERTEX_POINT ( 'NONE', #3359 ) ;
#4469=EDGE_CURVE ( 'NONE', #1957, #2969, #2541, .T. ) ;
#4470=DIRECTION ( 'NONE',  ( 0.000000000000000000, 0.000000000000000000, 1.000000000000000000 ) ) ;
#4473=ADVANCED_FACE ( 'NONE', ( #2565, #3642, #4360, #1831 ), #4107, .T. ) ;
#4476=ORIENTED_EDGE ( 'NONE', *, *, #3939, .T. ) ;
#4478=ORIENTED_EDGE ( 'NONE', *, *, #2139, .T. ) ;
#4484=VERTEX_POINT ( 'NONE', #3664 ) ;
#4487=ADVANCED_FACE ( 'NONE', ( #405 ), #2975, .F. ) ;
#4490=CARTESIAN_POINT ( 'NONE',  ( -2.644755406393140440, 29.88376691385261097, 5.987824696368042154 ) ) ;
#4492=CARTESIAN_POINT ( 'NONE',  ( -18.35933649373370358, 23.72646225117216900, 7.709376215153277201 ) ) ;
#4503=CARTESIAN_POINT ( 'NONE',  ( 26.00000000000000355, 3.184081677783117796E-15, 20.00001200000000168 ) ) ;
#4509=FACE_OUTER_BOUND ( 'NONE', #4606, .T. ) ;
#4510=LINE ( 'NONE', #4227, #2085 ) ;
#4515=CARTESIAN_POINT ( 'NONE',  ( 0.000000000000000000, 0.000000000000000000, 17.00000000000000000 ) ) ;
#4523=VERTEX_POINT ( 'NONE', #4431 ) ;
#4524=DIRECTION ( 'NONE',  ( 0.7071067811865462405, -0.7071067811865487940, 0.000000000000000000 ) ) ;
#4526=VECTOR ( 'NONE', #4222, 1000.000000000000000 ) ;
#4531=EDGE_CURVE ( 'NONE', #786, #2854, #4078, .T. ) ;
#4536=CARTESIAN_POINT ( 'NONE',  ( 18.21571070649545732, 23.83674813237291090, 9.520895848189299571 ) ) ;
#4538=CARTESIAN_POINT ( 'NONE',  ( 0.5000000000000001110, 10.00000000000000000, 13.00000000000000178 ) ) ;
#4540=CARTESIAN_POINT ( 'NONE',  ( 0.000000000000000000, 0.000000000000000000, 19.00000000000000000 ) ) ;
#4542=ORIENTED_EDGE ( 'NONE', *, *, #1586, .T. ) ;
#4545=AXIS2_PLACEMENT_3D ( 'NONE', #2666, #867, #2304 ) ;
#4547=CARTESIAN_POINT ( 'NONE',  ( 0.000000000000000000, 0.000000000000000000, 20.00000000000000000 ) ) ;
#4548=CARTESIAN_POINT ( 'NONE',  ( 0.000000000000000000, 10.00000000000000000, 15.00000000000000178 ) ) ;
#4560=EDGE_CURVE ( 'NONE', #4118, #4099, #2379, .T. ) ;
#4566=AXIS2_PLACEMENT_3D ( 'NONE', #930, #4569, #953 ) ;
#4569=DIRECTION ( 'NONE',  ( 0.7071067811865487940, -0.7071067811865463515, 0.000000000000000000 ) ) ;
#4571=AXIS2_PLACEMENT_3D ( 'NONE', #2582, #2653, #3038 ) ;
#4573=ORIENTED_EDGE ( 'NONE', *, *, #4339, .T. ) ;
#4576=LINE ( 'NONE', #2761, #4526 ) ;
#4581=DIRECTION ( 'NONE',  ( 1.000000000000000000, 0.000000000000000000, -0.000000000000000000 ) ) ;
#4582=CARTESIAN_POINT ( 'NONE',  ( 25.99307600111999150, -0.5999999999999998668, 20.00001200000000168 ) ) ;
#4586=LINE ( 'NONE', #2038, #3616 ) ;
#4587=EDGE_CURVE ( 'NONE', #3924, #1957, #3528, .T. ) ;
#4589=EDGE_CURVE ( 'NONE', #2288, #907, #2013, .T. ) ;
#4593=ORIENTED_EDGE ( 'NONE', *, *, #897, .T. ) ;
#4599=AXIS2_PLACEMENT_3D ( 'NONE', #3341, #1483, #1504 ) ;
#4601=PLANE ( 'NONE',  #3117 ) ;
#4606=EDGE_LOOP ( 'NONE', ( #284, #869 ) ) ;
#4610=CARTESIAN_POINT ( 'NONE',  ( -3.470226642398214878, 29.79897209676519765, 11.00633161724385900 ) ) ;
#4612=PRODUCT_DEFINITION_FORMATION_WITH_SPECIFIED_SOURCE ( 'ANY', '', #3774, .NOT_KNOWN. ) ;
#4619=ORIENTED_EDGE ( 'NONE', *, *, #2395, .F. ) ;
#4621=CARTESIAN_POINT ( 'NONE',  ( 0.000000000000000000, 0.000000000000000000, 19.00000000000000000 ) ) ;
#4625=( NAMED_UNIT ( * ) PLANE_ANGLE_UNIT ( ) SI_UNIT ( $, .RADIAN. ) );
#4628=DIRECTION ( 'NONE',  ( -0.000000000000000000, -0.000000000000000000, 1.000000000000000000 ) ) ;
#4631=CARTESIAN_POINT ( 'NONE',  ( 1.295195626368611075, 29.97299535330734699, 5.206545655307601272 ) ) ;
#4635=CARTESIAN_POINT ( 'NONE',  ( 23.52435923723758648, 18.61790092284045883, 11.00811882721853330 ) ) ;
#4637=FACE_OUTER_BOUND ( 'NONE', #4024, .T. ) ;
#4639=EDGE_CURVE ( 'NONE', #4523, #2288, #4576, .T. ) ;
#4647=CARTESIAN_POINT ( 'NONE',  ( 27.09999999999999787, 0.6000000000000000888, 19.00000000000000000 ) ) ;
#4648=DIRECTION ( 'NONE',  ( 0.000000000000000000, 0.000000000000000000, -1.000000000000000000 ) ) ;
#4649=CONICAL_SURFACE ( 'NONE', #1983, 27.99999999999999645, 0.7853981633974457255 ) ;
#4652=CARTESIAN_POINT ( 'NONE',  ( 24.67207871933482011, 8.377607117416825844, 20.00001200000000168 ) ) ;
#4655=ADVANCED_FACE ( 'NONE', ( #1575 ), #3025, .T. ) ;
#4657=CARTESIAN_POINT ( 'NONE',  ( 3.794405662118193856, 29.75924672568546114, 10.29276539630767573 ) ) ;
#4660=AXIS2_PLACEMENT_3D ( 'NONE', #2394, #2714, #2370 ) ;
#4664=CARTESIAN_POINT ( 'NONE',  ( 0.000000000000000000, 0.000000000000000000, 0.000000000000000000 ) ) ;
#4666=AXIS2_PLACEMENT_3D ( 'NONE', #3544, #4244, #1406 ) ;
#4676=CARTESIAN_POINT ( 'NONE',  ( -24.00000000000000355, 2.939152317953648289E-15, 17.00000000000000000 ) ) ;
#4679=CIRCLE ( 'NONE', #794, 30.00000000000000355 ) ;
#4681=CARTESIAN_POINT ( 'NONE',  ( 1.776153951180677870, 29.94834318124550165, 5.406519136333786335 ) ) ;
#4686=AXIS2_PLACEMENT_3D ( 'NONE', #2050, #241, #1691 ) ;
#4702=PLANE ( 'NONE',  #4666 ) ;
#4705=CARTESIAN_POINT ( 'NONE',  ( 0.5208970779615244018, 29.99659053120184282, 12.97467366945674172 ) ) ;
#4707=CARTESIAN_POINT ( 'NONE',  ( 24.00000000000000355, 0.000000000000000000, 19.00000000000000000 ) ) ;
#4730=COLOUR_RGB('Sky Blue',0.24,0.69,0.87);
#4731=FILL_AREA_STYLE_COLOUR('',#4730);
#4732=FILL_AREA_STYLE('',(#4731));
#4733=SURFACE_STYLE_FILL_AREA(#4732);
#4734=SURFACE_SIDE_STYLE('',(#4733));
#4735=SURFACE_STYLE_USAGE(.BOTH.,#4734);
#4736=PRESENTATION_STYLE_ASSIGNMENT((#4735));
ENDSEC;
END-ISO-10303-21;
